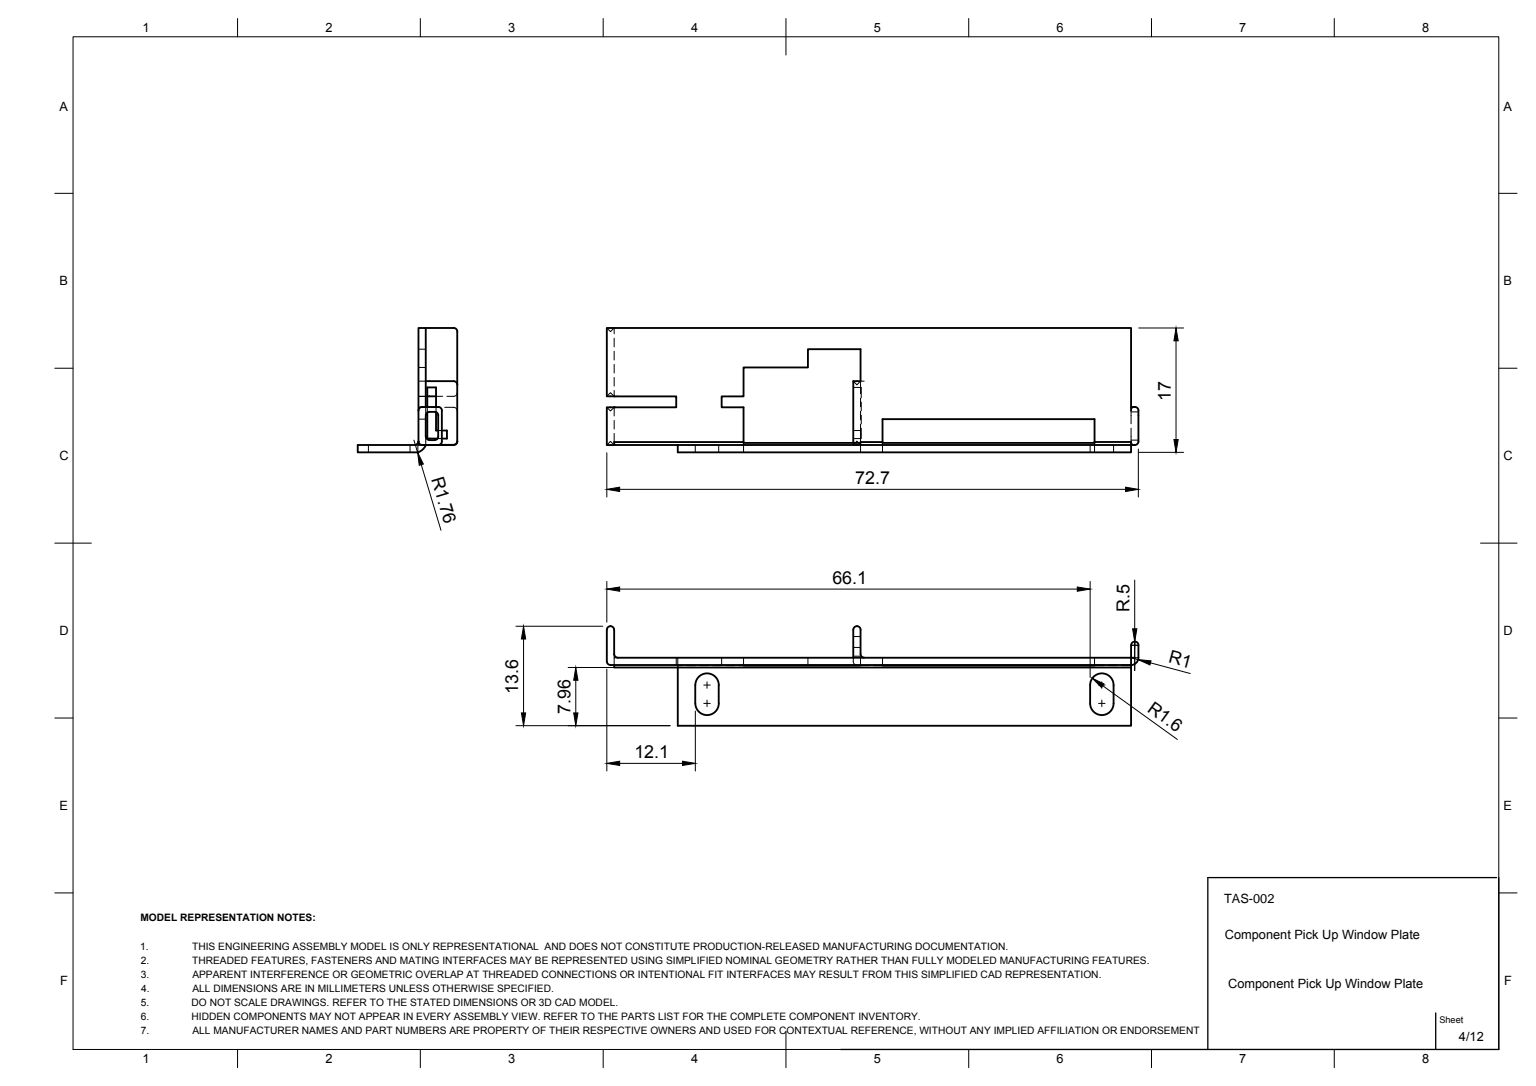
ISO-10303-21;
HEADER;
/* Generated by software containing ST-Developer
 * from STEP Tools, Inc. (www.steptools.com) 
 */

FILE_DESCRIPTION(
/* description */ ('STEP AP214'),
/* implementation_level */ '2;1');

FILE_NAME(
/* name */ 'Component Pick Up Window Plate.step',
/* time_stamp */ '2026-11-04T19:38:14-08:00',
/* author */ (''),
/* organization */ (''),
/* preprocessor_version */ 'ST-DEVELOPER v20.2',
/* originating_system */ 'Autodesk Translation Framework v15.17.0.0',
/* authorisation */ '');

FILE_SCHEMA (('AUTOMOTIVE_DESIGN { 1 0 10303 214 3 1 1 }'));
ENDSEC;

DATA;
#10=MECHANICAL_DESIGN_GEOMETRIC_PRESENTATION_REPRESENTATION('',(#471),#36668);
#385=SPHERICAL_SURFACE('',#18134,0.5);
#386=SPHERICAL_SURFACE('',#18138,0.5);
#407=(
BOUNDED_SURFACE()
B_SPLINE_SURFACE(2,2,((#25054,#25055,#25056),(#25057,#25058,#25059),(#25060,
#25061,#25062)),.UNSPECIFIED.,.F.,.F.,.F.)
B_SPLINE_SURFACE_WITH_KNOTS((3,3),(3,3),(-1.57079632679491,1.51262184115385E-31),
(-3.14159265358979,-1.57079632679489),.UNSPECIFIED.)
GEOMETRIC_REPRESENTATION_ITEM()
RATIONAL_B_SPLINE_SURFACE(((1.,0.707106781186547,1.),(0.707106781186636,
0.500000000000062,0.707106781186636),(1.,0.707106781186547,1.)))
REPRESENTATION_ITEM('')
SURFACE()
);
#408=(
BOUNDED_SURFACE()
B_SPLINE_SURFACE(2,2,((#25105,#25106,#25107),(#25108,#25109,#25110),(#25111,
#25112,#25113)),.UNSPECIFIED.,.F.,.F.,.F.)
B_SPLINE_SURFACE_WITH_KNOTS((3,3),(3,3),(-1.5707963267949,4.00000000000002E-15),
(-1.5707963267949,8.88178419700128E-15),.UNSPECIFIED.)
GEOMETRIC_REPRESENTATION_ITEM()
RATIONAL_B_SPLINE_SURFACE(((1.,0.707106781186544,1.),(0.707106781186621,
0.50000000000005,0.707106781186621),(1.,0.707106781186544,1.)))
REPRESENTATION_ITEM('')
SURFACE()
);
#417=ELLIPSE('',#18107,0.707106781183618,0.499999999997816);
#418=ELLIPSE('',#18108,0.70710678118541,0.499999999999275);
#419=ELLIPSE('',#18109,0.707106781187129,0.500000000000412);
#420=ELLIPSE('',#18110,0.707106781186662,0.500000000000074);
#421=ELLIPSE('',#18114,0.707106781185328,0.499999999999127);
#422=ELLIPSE('',#18115,0.707106781186805,0.500000000000239);
#423=ELLIPSE('',#18116,0.707106781186168,0.499999999999746);
#424=ELLIPSE('',#18117,0.707106781186428,0.499999999999895);
#425=ELLIPSE('',#18121,0.707106781186371,0.500000000000029);
#426=ELLIPSE('',#18122,0.707106781185591,0.499999999999375);
#427=ELLIPSE('',#18123,0.707106781187582,0.500000000000786);
#428=ELLIPSE('',#18124,0.707106781187168,0.500000000000398);
#451=SHAPE_REPRESENTATION_RELATIONSHIP('SRR','None',#36707,#461);
#461=ADVANCED_BREP_SHAPE_REPRESENTATION('',(#481),#36659);
#471=STYLED_ITEM('',(#36766),#481);
#481=MANIFOLD_SOLID_BREP('Body1',#17794);
#515=CYLINDRICAL_SURFACE('',#18106,0.5);
#516=CYLINDRICAL_SURFACE('',#18111,0.5);
#517=CYLINDRICAL_SURFACE('',#18112,0.5);
#518=CYLINDRICAL_SURFACE('',#18113,0.5);
#519=CYLINDRICAL_SURFACE('',#18118,0.5);
#520=CYLINDRICAL_SURFACE('',#18119,0.5);
#521=CYLINDRICAL_SURFACE('',#18120,0.5);
#522=CYLINDRICAL_SURFACE('',#18125,0.5);
#523=CYLINDRICAL_SURFACE('',#18126,0.5);
#524=CYLINDRICAL_SURFACE('',#18131,0.5);
#525=CYLINDRICAL_SURFACE('',#18136,0.5);
#526=CYLINDRICAL_SURFACE('',#18140,0.5);
#527=CYLINDRICAL_SURFACE('',#18147,0.5);
#528=CYLINDRICAL_SURFACE('',#18157,0.5);
#529=CYLINDRICAL_SURFACE('',#18160,0.5);
#530=CYLINDRICAL_SURFACE('',#18167,0.5);
#531=CYLINDRICAL_SURFACE('',#18170,0.5);
#532=CYLINDRICAL_SURFACE('',#18173,0.5);
#533=CYLINDRICAL_SURFACE('',#18176,0.5);
#534=CYLINDRICAL_SURFACE('',#18197,0.5);
#535=CYLINDRICAL_SURFACE('',#18200,0.5);
#536=CYLINDRICAL_SURFACE('',#18203,0.5);
#537=CYLINDRICAL_SURFACE('',#18206,0.5);
#538=CYLINDRICAL_SURFACE('',#18209,1.);
#539=CYLINDRICAL_SURFACE('',#18231,1.6);
#540=CYLINDRICAL_SURFACE('',#18235,1.6);
#541=CYLINDRICAL_SURFACE('',#18239,1.6);
#542=CYLINDRICAL_SURFACE('',#18243,1.6);
#543=CYLINDRICAL_SURFACE('',#18253,2.15235845279182);
#544=CYLINDRICAL_SURFACE('',#18258,1.76114216495771);
#545=CYLINDRICAL_SURFACE('',#18261,1.76114216495771);
#546=CYLINDRICAL_SURFACE('',#18262,1.76114216495771);
#880=FACE_BOUND('',#2725,.T.);
#881=FACE_BOUND('',#2780,.T.);
#882=FACE_BOUND('',#2781,.T.);
#883=FACE_BOUND('',#2788,.T.);
#884=FACE_BOUND('',#2789,.T.);
#1025=CIRCLE('',#18127,0.5);
#1026=CIRCLE('',#18128,1.);
#1027=CIRCLE('',#18129,0.5);
#1028=CIRCLE('',#18130,0.5);
#1029=CIRCLE('',#18132,0.5);
#1030=CIRCLE('',#18133,0.5);
#1031=CIRCLE('',#18135,0.5);
#1032=CIRCLE('',#18137,0.5);
#1033=CIRCLE('',#18139,0.5);
#1034=CIRCLE('',#18141,0.5);
#1035=CIRCLE('',#18142,0.5);
#1036=CIRCLE('',#18143,0.5);
#1037=CIRCLE('',#18144,0.5);
#1038=CIRCLE('',#18145,0.5);
#1039=CIRCLE('',#18146,1.);
#1040=CIRCLE('',#18148,0.5);
#1041=CIRCLE('',#18150,0.5);
#1042=CIRCLE('',#18155,0.5);
#1043=CIRCLE('',#18158,0.5);
#1044=CIRCLE('',#18159,0.5);
#1045=CIRCLE('',#18161,0.5);
#1046=CIRCLE('',#18162,0.5);
#1047=CIRCLE('',#18168,0.5);
#1048=CIRCLE('',#18169,0.5);
#1049=CIRCLE('',#18171,0.5);
#1050=CIRCLE('',#18172,0.5);
#1051=CIRCLE('',#18174,0.5);
#1052=CIRCLE('',#18175,0.5);
#1053=CIRCLE('',#18177,0.5);
#1054=CIRCLE('',#18178,0.5);
#1055=CIRCLE('',#18198,0.5);
#1056=CIRCLE('',#18199,0.5);
#1057=CIRCLE('',#18201,0.5);
#1058=CIRCLE('',#18202,0.5);
#1059=CIRCLE('',#18204,0.5);
#1060=CIRCLE('',#18205,0.5);
#1061=CIRCLE('',#18207,0.5);
#1062=CIRCLE('',#18208,0.5);
#1063=CIRCLE('',#18219,1.76114216495771);
#1064=CIRCLE('',#18220,2.15235845279182);
#1065=CIRCLE('',#18222,2.15235845279183);
#1066=CIRCLE('',#18223,1.76114216495771);
#1067=CIRCLE('',#18226,1.76114216495771);
#1068=CIRCLE('',#18227,2.15235845279182);
#1069=CIRCLE('',#18229,1.76114216495771);
#1070=CIRCLE('',#18230,2.15235845279182);
#1071=CIRCLE('',#18232,1.6);
#1072=CIRCLE('',#18233,1.6);
#1073=CIRCLE('',#18236,1.6);
#1074=CIRCLE('',#18237,1.6);
#1075=CIRCLE('',#18240,1.6);
#1076=CIRCLE('',#18241,1.6);
#1077=CIRCLE('',#18244,1.6);
#1078=CIRCLE('',#18245,1.6);
#1079=CIRCLE('',#18248,1.76114216495771);
#1080=CIRCLE('',#18251,2.15235845279182);
#1081=CIRCLE('',#18254,2.15235845279182);
#1082=CIRCLE('',#18263,1.76114216495771);
#1663=FACE_OUTER_BOUND('',#2698,.T.);
#1664=FACE_OUTER_BOUND('',#2699,.T.);
#1665=FACE_OUTER_BOUND('',#2700,.T.);
#1666=FACE_OUTER_BOUND('',#2701,.T.);
#1667=FACE_OUTER_BOUND('',#2702,.T.);
#1668=FACE_OUTER_BOUND('',#2703,.T.);
#1669=FACE_OUTER_BOUND('',#2704,.T.);
#1670=FACE_OUTER_BOUND('',#2705,.T.);
#1671=FACE_OUTER_BOUND('',#2706,.T.);
#1672=FACE_OUTER_BOUND('',#2707,.T.);
#1673=FACE_OUTER_BOUND('',#2708,.T.);
#1674=FACE_OUTER_BOUND('',#2709,.T.);
#1675=FACE_OUTER_BOUND('',#2710,.T.);
#1676=FACE_OUTER_BOUND('',#2711,.T.);
#1677=FACE_OUTER_BOUND('',#2712,.T.);
#1678=FACE_OUTER_BOUND('',#2713,.T.);
#1679=FACE_OUTER_BOUND('',#2714,.T.);
#1680=FACE_OUTER_BOUND('',#2715,.T.);
#1681=FACE_OUTER_BOUND('',#2716,.T.);
#1682=FACE_OUTER_BOUND('',#2717,.T.);
#1683=FACE_OUTER_BOUND('',#2718,.T.);
#1684=FACE_OUTER_BOUND('',#2719,.T.);
#1685=FACE_OUTER_BOUND('',#2720,.T.);
#1686=FACE_OUTER_BOUND('',#2721,.T.);
#1687=FACE_OUTER_BOUND('',#2722,.T.);
#1688=FACE_OUTER_BOUND('',#2723,.T.);
#1689=FACE_OUTER_BOUND('',#2724,.T.);
#1690=FACE_OUTER_BOUND('',#2726,.T.);
#1691=FACE_OUTER_BOUND('',#2727,.T.);
#1692=FACE_OUTER_BOUND('',#2728,.T.);
#1693=FACE_OUTER_BOUND('',#2729,.T.);
#1694=FACE_OUTER_BOUND('',#2730,.T.);
#1695=FACE_OUTER_BOUND('',#2731,.T.);
#1696=FACE_OUTER_BOUND('',#2732,.T.);
#1697=FACE_OUTER_BOUND('',#2733,.T.);
#1698=FACE_OUTER_BOUND('',#2734,.T.);
#1699=FACE_OUTER_BOUND('',#2735,.T.);
#1700=FACE_OUTER_BOUND('',#2736,.T.);
#1701=FACE_OUTER_BOUND('',#2737,.T.);
#1702=FACE_OUTER_BOUND('',#2738,.T.);
#1703=FACE_OUTER_BOUND('',#2739,.T.);
#1704=FACE_OUTER_BOUND('',#2740,.T.);
#1705=FACE_OUTER_BOUND('',#2741,.T.);
#1706=FACE_OUTER_BOUND('',#2742,.T.);
#1707=FACE_OUTER_BOUND('',#2743,.T.);
#1708=FACE_OUTER_BOUND('',#2744,.T.);
#1709=FACE_OUTER_BOUND('',#2745,.T.);
#1710=FACE_OUTER_BOUND('',#2746,.T.);
#1711=FACE_OUTER_BOUND('',#2747,.T.);
#1712=FACE_OUTER_BOUND('',#2748,.T.);
#1713=FACE_OUTER_BOUND('',#2749,.T.);
#1714=FACE_OUTER_BOUND('',#2750,.T.);
#1715=FACE_OUTER_BOUND('',#2751,.T.);
#1716=FACE_OUTER_BOUND('',#2752,.T.);
#1717=FACE_OUTER_BOUND('',#2753,.T.);
#1718=FACE_OUTER_BOUND('',#2754,.T.);
#1719=FACE_OUTER_BOUND('',#2755,.T.);
#1720=FACE_OUTER_BOUND('',#2756,.T.);
#1721=FACE_OUTER_BOUND('',#2757,.T.);
#1722=FACE_OUTER_BOUND('',#2758,.T.);
#1723=FACE_OUTER_BOUND('',#2759,.T.);
#1724=FACE_OUTER_BOUND('',#2760,.T.);
#1725=FACE_OUTER_BOUND('',#2761,.T.);
#1726=FACE_OUTER_BOUND('',#2762,.T.);
#1727=FACE_OUTER_BOUND('',#2763,.T.);
#1728=FACE_OUTER_BOUND('',#2764,.T.);
#1729=FACE_OUTER_BOUND('',#2765,.T.);
#1730=FACE_OUTER_BOUND('',#2766,.T.);
#1731=FACE_OUTER_BOUND('',#2767,.T.);
#1732=FACE_OUTER_BOUND('',#2768,.T.);
#1733=FACE_OUTER_BOUND('',#2769,.T.);
#1734=FACE_OUTER_BOUND('',#2770,.T.);
#1735=FACE_OUTER_BOUND('',#2771,.T.);
#1736=FACE_OUTER_BOUND('',#2772,.T.);
#1737=FACE_OUTER_BOUND('',#2773,.T.);
#1738=FACE_OUTER_BOUND('',#2774,.T.);
#1739=FACE_OUTER_BOUND('',#2775,.T.);
#1740=FACE_OUTER_BOUND('',#2776,.T.);
#1741=FACE_OUTER_BOUND('',#2777,.T.);
#1742=FACE_OUTER_BOUND('',#2778,.T.);
#1743=FACE_OUTER_BOUND('',#2779,.T.);
#1744=FACE_OUTER_BOUND('',#2782,.T.);
#1745=FACE_OUTER_BOUND('',#2783,.T.);
#1746=FACE_OUTER_BOUND('',#2784,.T.);
#1747=FACE_OUTER_BOUND('',#2785,.T.);
#1748=FACE_OUTER_BOUND('',#2786,.T.);
#1749=FACE_OUTER_BOUND('',#2787,.T.);
#1750=FACE_OUTER_BOUND('',#2790,.T.);
#1751=FACE_OUTER_BOUND('',#2791,.T.);
#1752=FACE_OUTER_BOUND('',#2792,.T.);
#1753=FACE_OUTER_BOUND('',#2793,.T.);
#1754=FACE_OUTER_BOUND('',#2794,.T.);
#1755=FACE_OUTER_BOUND('',#2795,.T.);
#1756=FACE_OUTER_BOUND('',#2796,.T.);
#1757=FACE_OUTER_BOUND('',#2797,.T.);
#1758=FACE_OUTER_BOUND('',#2798,.T.);
#2698=EDGE_LOOP('',(#12018,#12019,#12020,#12021,#12022,#12023));
#2699=EDGE_LOOP('',(#12024,#12025,#12026));
#2700=EDGE_LOOP('',(#12027,#12028,#12029));
#2701=EDGE_LOOP('',(#12030,#12031,#12032,#12033,#12034,#12035));
#2702=EDGE_LOOP('',(#12036,#12037,#12038));
#2703=EDGE_LOOP('',(#12039,#12040,#12041));
#2704=EDGE_LOOP('',(#12042,#12043,#12044,#12045,#12046,#12047));
#2705=EDGE_LOOP('',(#12048,#12049,#12050));
#2706=EDGE_LOOP('',(#12051,#12052,#12053));
#2707=EDGE_LOOP('',(#12054,#12055,#12056,#12057));
#2708=EDGE_LOOP('',(#12058,#12059,#12060,#12061,#12062));
#2709=EDGE_LOOP('',(#12063,#12064));
#2710=EDGE_LOOP('',(#12065,#12066,#12067,#12068,#12069,#12070,#12071,#12072));
#2711=EDGE_LOOP('',(#12073,#12074));
#2712=EDGE_LOOP('',(#12075,#12076,#12077,#12078,#12079));
#2713=EDGE_LOOP('',(#12080,#12081,#12082,#12083,#12084));
#2714=EDGE_LOOP('',(#12085,#12086,#12087,#12088));
#2715=EDGE_LOOP('',(#12089,#12090,#12091,#12092,#12093));
#2716=EDGE_LOOP('',(#12094,#12095,#12096,#12097));
#2717=EDGE_LOOP('',(#12098,#12099,#12100,#12101));
#2718=EDGE_LOOP('',(#12102,#12103,#12104,#12105));
#2719=EDGE_LOOP('',(#12106,#12107,#12108,#12109,#12110));
#2720=EDGE_LOOP('',(#12111,#12112,#12113,#12114));
#2721=EDGE_LOOP('',(#12115,#12116,#12117,#12118));
#2722=EDGE_LOOP('',(#12119,#12120,#12121,#12122,#12123,#12124,#12125,#12126));
#2723=EDGE_LOOP('',(#12127,#12128,#12129,#12130,#12131,#12132,#12133,#12134));
#2724=EDGE_LOOP('',(#12135,#12136,#12137,#12138));
#2725=EDGE_LOOP('',(#12139,#12140,#12141,#12142,#12143,#12144));
#2726=EDGE_LOOP('',(#12145,#12146,#12147,#12148,#12149,#12150,#12151,#12152));
#2727=EDGE_LOOP('',(#12153,#12154,#12155,#12156,#12157,#12158,#12159,#12160,
#12161,#12162));
#2728=EDGE_LOOP('',(#12163,#12164,#12165,#12166));
#2729=EDGE_LOOP('',(#12167,#12168,#12169,#12170));
#2730=EDGE_LOOP('',(#12171,#12172,#12173,#12174));
#2731=EDGE_LOOP('',(#12175,#12176,#12177,#12178));
#2732=EDGE_LOOP('',(#12179,#12180,#12181,#12182));
#2733=EDGE_LOOP('',(#12183,#12184,#12185,#12186));
#2734=EDGE_LOOP('',(#12187,#12188,#12189,#12190));
#2735=EDGE_LOOP('',(#12191,#12192,#12193,#12194));
#2736=EDGE_LOOP('',(#12195,#12196,#12197,#12198));
#2737=EDGE_LOOP('',(#12199,#12200,#12201,#12202));
#2738=EDGE_LOOP('',(#12203,#12204,#12205,#12206));
#2739=EDGE_LOOP('',(#12207,#12208,#12209,#12210));
#2740=EDGE_LOOP('',(#12211,#12212,#12213,#12214));
#2741=EDGE_LOOP('',(#12215,#12216,#12217,#12218,#12219));
#2742=EDGE_LOOP('',(#12220,#12221,#12222,#12223));
#2743=EDGE_LOOP('',(#12224,#12225,#12226,#12227));
#2744=EDGE_LOOP('',(#12228,#12229,#12230,#12231));
#2745=EDGE_LOOP('',(#12232,#12233,#12234,#12235,#12236,#12237,#12238,#12239));
#2746=EDGE_LOOP('',(#12240,#12241,#12242,#12243,#12244));
#2747=EDGE_LOOP('',(#12245,#12246,#12247,#12248));
#2748=EDGE_LOOP('',(#12249,#12250,#12251,#12252,#12253));
#2749=EDGE_LOOP('',(#12254,#12255,#12256,#12257,#12258,#12259,#12260,#12261));
#2750=EDGE_LOOP('',(#12262,#12263,#12264,#12265));
#2751=EDGE_LOOP('',(#12266,#12267,#12268,#12269));
#2752=EDGE_LOOP('',(#12270,#12271,#12272,#12273));
#2753=EDGE_LOOP('',(#12274,#12275,#12276,#12277));
#2754=EDGE_LOOP('',(#12278,#12279,#12280,#12281,#12282,#12283));
#2755=EDGE_LOOP('',(#12284,#12285,#12286,#12287));
#2756=EDGE_LOOP('',(#12288,#12289,#12290,#12291));
#2757=EDGE_LOOP('',(#12292,#12293,#12294,#12295));
#2758=EDGE_LOOP('',(#12296,#12297,#12298,#12299,#12300,#12301));
#2759=EDGE_LOOP('',(#12302,#12303,#12304,#12305,#12306,#12307));
#2760=EDGE_LOOP('',(#12308,#12309,#12310));
#2761=EDGE_LOOP('',(#12311,#12312,#12313));
#2762=EDGE_LOOP('',(#12314,#12315,#12316,#12317));
#2763=EDGE_LOOP('',(#12318,#12319,#12320,#12321,#12322,#12323));
#2764=EDGE_LOOP('',(#12324,#12325,#12326,#12327,#12328,#12329,#12330));
#2765=EDGE_LOOP('',(#12331,#12332,#12333,#12334));
#2766=EDGE_LOOP('',(#12335,#12336,#12337,#12338,#12339,#12340));
#2767=EDGE_LOOP('',(#12341,#12342,#12343,#12344,#12345,#12346));
#2768=EDGE_LOOP('',(#12347,#12348,#12349,#12350));
#2769=EDGE_LOOP('',(#12351,#12352,#12353,#12354));
#2770=EDGE_LOOP('',(#12355,#12356,#12357,#12358));
#2771=EDGE_LOOP('',(#12359,#12360,#12361,#12362));
#2772=EDGE_LOOP('',(#12363,#12364,#12365,#12366));
#2773=EDGE_LOOP('',(#12367,#12368,#12369,#12370));
#2774=EDGE_LOOP('',(#12371,#12372,#12373,#12374));
#2775=EDGE_LOOP('',(#12375,#12376,#12377,#12378));
#2776=EDGE_LOOP('',(#12379,#12380,#12381,#12382,#12383));
#2777=EDGE_LOOP('',(#12384,#12385,#12386,#12387,#12388,#12389));
#2778=EDGE_LOOP('',(#12390,#12391,#12392));
#2779=EDGE_LOOP('',(#12393,#12394,#12395,#12396));
#2780=EDGE_LOOP('',(#12397,#12398,#12399,#12400));
#2781=EDGE_LOOP('',(#12401,#12402,#12403,#12404));
#2782=EDGE_LOOP('',(#12405,#12406,#12407,#12408,#12409,#12410,#12411,#12412,
#12413,#12414,#12415,#12416,#12417));
#2783=EDGE_LOOP('',(#12418,#12419,#12420,#12421,#12422,#12423,#12424,#12425,
#12426,#12427,#12428,#12429,#12430,#12431,#12432,#12433,#12434,#12435,#12436,
#12437,#12438,#12439,#12440,#12441,#12442,#12443,#12444,#12445,#12446,#12447,
#12448,#12449,#12450,#12451));
#2784=EDGE_LOOP('',(#12452,#12453,#12454,#12455,#12456,#12457,#12458,#12459));
#2785=EDGE_LOOP('',(#12460,#12461,#12462,#12463,#12464,#12465,#12466,#12467,
#12468,#12469,#12470,#12471,#12472,#12473,#12474,#12475,#12476,#12477,#12478,
#12479,#12480,#12481,#12482,#12483,#12484,#12485,#12486,#12487,#12488,#12489,
#12490,#12491,#12492,#12493,#12494,#12495,#12496,#12497));
#2786=EDGE_LOOP('',(#12498,#12499,#12500,#12501));
#2787=EDGE_LOOP('',(#12502,#12503,#12504,#12505,#12506,#12507,#12508,#12509));
#2788=EDGE_LOOP('',(#12510,#12511,#12512,#12513));
#2789=EDGE_LOOP('',(#12514,#12515,#12516,#12517));
#2790=EDGE_LOOP('',(#12518,#12519,#12520,#12521));
#2791=EDGE_LOOP('',(#12522,#12523,#12524,#12525));
#2792=EDGE_LOOP('',(#12526,#12527,#12528,#12529));
#2793=EDGE_LOOP('',(#12530,#12531,#12532,#12533,#12534,#12535,#12536));
#2794=EDGE_LOOP('',(#12537,#12538,#12539,#12540,#12541));
#2795=EDGE_LOOP('',(#12542,#12543,#12544,#12545));
#2796=EDGE_LOOP('',(#12546,#12547,#12548,#12549));
#2797=EDGE_LOOP('',(#12550,#12551,#12552,#12553,#12554,#12555));
#2798=EDGE_LOOP('',(#12556,#12557,#12558,#12559,#12560,#12561));
#3936=LINE('',#25010,#5646);
#3937=LINE('',#25015,#5647);
#3938=LINE('',#25017,#5648);
#3939=LINE('',#25019,#5649);
#3940=LINE('',#25027,#5650);
#3941=LINE('',#25032,#5651);
#3942=LINE('',#25034,#5652);
#3943=LINE('',#25036,#5653);
#3944=LINE('',#25044,#5654);
#3945=LINE('',#25049,#5655);
#3946=LINE('',#25051,#5656);
#3947=LINE('',#25053,#5657);
#3948=LINE('',#25076,#5658);
#3949=LINE('',#25078,#5659);
#3950=LINE('',#25086,#5660);
#3951=LINE('',#25088,#5661);
#3952=LINE('',#25089,#5662);
#3953=LINE('',#25091,#5663);
#3954=LINE('',#25093,#5664);
#3955=LINE('',#25094,#5665);
#3956=LINE('',#25103,#5666);
#3957=LINE('',#25104,#5667);
#3958=LINE('',#25123,#5668);
#3959=LINE('',#25125,#5669);
#3960=LINE('',#25130,#5670);
#3961=LINE('',#25134,#5671);
#3962=LINE('',#25136,#5672);
#3963=LINE('',#25137,#5673);
#3964=LINE('',#25140,#5674);
#3965=LINE('',#25142,#5675);
#3966=LINE('',#25143,#5676);
#3967=LINE('',#25146,#5677);
#3968=LINE('',#25148,#5678);
#3969=LINE('',#25149,#5679);
#3970=LINE('',#25152,#5680);
#3971=LINE('',#25154,#5681);
#3972=LINE('',#25155,#5682);
#3973=LINE('',#25158,#5683);
#3974=LINE('',#25160,#5684);
#3975=LINE('',#25162,#5685);
#3976=LINE('',#25165,#5686);
#3977=LINE('',#25166,#5687);
#3978=LINE('',#25172,#5688);
#3979=LINE('',#25175,#5689);
#3980=LINE('',#25178,#5690);
#3981=LINE('',#25180,#5691);
#3982=LINE('',#25184,#5692);
#3983=LINE('',#25187,#5693);
#3984=LINE('',#25188,#5694);
#3985=LINE('',#25190,#5695);
#3986=LINE('',#25192,#5696);
#3987=LINE('',#25193,#5697);
#3988=LINE('',#25195,#5698);
#3989=LINE('',#25197,#5699);
#3990=LINE('',#25199,#5700);
#3991=LINE('',#25201,#5701);
#3992=LINE('',#25202,#5702);
#3993=LINE('',#25209,#5703);
#3994=LINE('',#25212,#5704);
#3995=LINE('',#25218,#5705);
#3996=LINE('',#25221,#5706);
#3997=LINE('',#25227,#5707);
#3998=LINE('',#25230,#5708);
#3999=LINE('',#25236,#5709);
#4000=LINE('',#25239,#5710);
#4001=LINE('',#25243,#5711);
#4002=LINE('',#25245,#5712);
#4003=LINE('',#25247,#5713);
#4004=LINE('',#25248,#5714);
#4005=LINE('',#25251,#5715);
#4006=LINE('',#25253,#5716);
#4007=LINE('',#25254,#5717);
#4008=LINE('',#25257,#5718);
#4009=LINE('',#25259,#5719);
#4010=LINE('',#25260,#5720);
#4011=LINE('',#25263,#5721);
#4012=LINE('',#25265,#5722);
#4013=LINE('',#25266,#5723);
#4014=LINE('',#25269,#5724);
#4015=LINE('',#25271,#5725);
#4016=LINE('',#25272,#5726);
#4017=LINE('',#25275,#5727);
#4018=LINE('',#25277,#5728);
#4019=LINE('',#25278,#5729);
#4020=LINE('',#25281,#5730);
#4021=LINE('',#25283,#5731);
#4022=LINE('',#25284,#5732);
#4023=LINE('',#25288,#5733);
#4024=LINE('',#25290,#5734);
#4025=LINE('',#25292,#5735);
#4026=LINE('',#25293,#5736);
#4027=LINE('',#25297,#5737);
#4028=LINE('',#25299,#5738);
#4029=LINE('',#25301,#5739);
#4030=LINE('',#25302,#5740);
#4031=LINE('',#25305,#5741);
#4032=LINE('',#25306,#5742);
#4033=LINE('',#25307,#5743);
#4034=LINE('',#25310,#5744);
#4035=LINE('',#25312,#5745);
#4036=LINE('',#25313,#5746);
#4037=LINE('',#25315,#5747);
#4038=LINE('',#25316,#5748);
#4039=LINE('',#25318,#5749);
#4040=LINE('',#25319,#5750);
#4041=LINE('',#25322,#5751);
#4042=LINE('',#25324,#5752);
#4043=LINE('',#25325,#5753);
#4044=LINE('',#25328,#5754);
#4045=LINE('',#25329,#5755);
#4046=LINE('',#25330,#5756);
#4047=LINE('',#25332,#5757);
#4048=LINE('',#25335,#5758);
#4049=LINE('',#25336,#5759);
#4050=LINE('',#25338,#5760);
#4051=LINE('',#25340,#5761);
#4052=LINE('',#25341,#5762);
#4053=LINE('',#25347,#5763);
#4054=LINE('',#25350,#5764);
#4055=LINE('',#25356,#5765);
#4056=LINE('',#25359,#5766);
#4057=LINE('',#25364,#5767);
#4058=LINE('',#25366,#5768);
#4059=LINE('',#25370,#5769);
#4060=LINE('',#25373,#5770);
#4061=LINE('',#25375,#5771);
#4062=LINE('',#25376,#5772);
#4063=LINE('',#25377,#5773);
#4064=LINE('',#25378,#5774);
#4065=LINE('',#25380,#5775);
#4066=LINE('',#25381,#5776);
#4067=LINE('',#25384,#5777);
#4068=LINE('',#25385,#5778);
#4069=LINE('',#25387,#5779);
#4070=LINE('',#25391,#5780);
#4071=LINE('',#25392,#5781);
#4072=LINE('',#25395,#5782);
#4073=LINE('',#25396,#5783);
#4074=LINE('',#25400,#5784);
#4075=LINE('',#25402,#5785);
#4076=LINE('',#25404,#5786);
#4077=LINE('',#25405,#5787);
#4078=LINE('',#25409,#5788);
#4079=LINE('',#25411,#5789);
#4080=LINE('',#25415,#5790);
#4081=LINE('',#25417,#5791);
#4082=LINE('',#25422,#5792);
#4083=LINE('',#25424,#5793);
#4084=LINE('',#25426,#5794);
#4085=LINE('',#25427,#5795);
#4086=LINE('',#25431,#5796);
#4087=LINE('',#25433,#5797);
#4088=LINE('',#25437,#5798);
#4089=LINE('',#25439,#5799);
#4090=LINE('',#25445,#5800);
#4091=LINE('',#25449,#5801);
#4092=LINE('',#25454,#5802);
#4093=LINE('',#25455,#5803);
#4094=LINE('',#25456,#5804);
#4095=LINE('',#25460,#5805);
#4096=LINE('',#25464,#5806);
#4097=LINE('',#25465,#5807);
#4098=LINE('',#25469,#5808);
#4099=LINE('',#25473,#5809);
#4100=LINE('',#25478,#5810);
#4101=LINE('',#25479,#5811);
#4102=LINE('',#25480,#5812);
#4103=LINE('',#25484,#5813);
#4104=LINE('',#25488,#5814);
#4105=LINE('',#25489,#5815);
#4106=LINE('',#25495,#5816);
#4107=LINE('',#25497,#5817);
#4108=LINE('',#25499,#5818);
#4109=LINE('',#25500,#5819);
#4110=LINE('',#25502,#5820);
#4111=LINE('',#25504,#5821);
#4112=LINE('',#25505,#5822);
#4113=LINE('',#25508,#5823);
#4114=LINE('',#25512,#5824);
#4115=LINE('',#25514,#5825);
#4116=LINE('',#25515,#5826);
#4117=LINE('',#25517,#5827);
#4118=LINE('',#25518,#5828);
#4119=LINE('',#25522,#5829);
#4120=LINE('',#25523,#5830);
#4121=LINE('',#25524,#5831);
#4122=LINE('',#25525,#5832);
#4123=LINE('',#25528,#5833);
#4124=LINE('',#25529,#5834);
#4125=LINE('',#25531,#5835);
#4126=LINE('',#25532,#5836);
#4127=LINE('',#25533,#5837);
#4128=LINE('',#25534,#5838);
#4129=LINE('',#25535,#5839);
#4130=LINE('',#25536,#5840);
#4131=LINE('',#25537,#5841);
#4132=LINE('',#25539,#5842);
#4133=LINE('',#25541,#5843);
#4134=LINE('',#25543,#5844);
#4135=LINE('',#25545,#5845);
#4136=LINE('',#25546,#5846);
#4137=LINE('',#25548,#5847);
#5646=VECTOR('',#20176,1000.);
#5647=VECTOR('',#20181,1000.);
#5648=VECTOR('',#20184,1000.);
#5649=VECTOR('',#20187,1000.);
#5650=VECTOR('',#20194,1000.);
#5651=VECTOR('',#20199,1000.);
#5652=VECTOR('',#20202,1000.);
#5653=VECTOR('',#20205,1000.);
#5654=VECTOR('',#20212,1000.);
#5655=VECTOR('',#20217,1000.);
#5656=VECTOR('',#20220,1000.);
#5657=VECTOR('',#20223,1000.);
#5658=VECTOR('',#20236,1000.);
#5659=VECTOR('',#20239,1000.);
#5660=VECTOR('',#20248,1000.);
#5661=VECTOR('',#20249,1000.);
#5662=VECTOR('',#20250,1000.);
#5663=VECTOR('',#20251,1000.);
#5664=VECTOR('',#20252,1000.);
#5665=VECTOR('',#20253,1000.);
#5666=VECTOR('',#20264,1000.);
#5667=VECTOR('',#20265,1000.);
#5668=VECTOR('',#20276,1000.);
#5669=VECTOR('',#20277,1000.);
#5670=VECTOR('',#20282,1000.);
#5671=VECTOR('',#20285,1000.);
#5672=VECTOR('',#20286,1000.);
#5673=VECTOR('',#20287,1000.);
#5674=VECTOR('',#20290,1000.);
#5675=VECTOR('',#20291,1000.);
#5676=VECTOR('',#20292,1000.);
#5677=VECTOR('',#20295,1000.);
#5678=VECTOR('',#20296,1000.);
#5679=VECTOR('',#20297,1000.);
#5680=VECTOR('',#20300,1000.);
#5681=VECTOR('',#20301,1000.);
#5682=VECTOR('',#20302,1000.);
#5683=VECTOR('',#20305,1000.);
#5684=VECTOR('',#20306,1000.);
#5685=VECTOR('',#20307,1000.);
#5686=VECTOR('',#20312,1000.);
#5687=VECTOR('',#20313,1000.);
#5688=VECTOR('',#20318,1000.);
#5689=VECTOR('',#20321,1000.);
#5690=VECTOR('',#20324,1000.);
#5691=VECTOR('',#20325,1000.);
#5692=VECTOR('',#20328,1000.);
#5693=VECTOR('',#20333,1000.);
#5694=VECTOR('',#20334,1000.);
#5695=VECTOR('',#20335,1000.);
#5696=VECTOR('',#20336,1000.);
#5697=VECTOR('',#20337,1000.);
#5698=VECTOR('',#20340,1000.);
#5699=VECTOR('',#20343,1000.);
#5700=VECTOR('',#20344,1000.);
#5701=VECTOR('',#20345,1000.);
#5702=VECTOR('',#20346,1000.);
#5703=VECTOR('',#20353,1000.);
#5704=VECTOR('',#20356,1000.);
#5705=VECTOR('',#20361,1000.);
#5706=VECTOR('',#20364,1000.);
#5707=VECTOR('',#20369,1000.);
#5708=VECTOR('',#20372,1000.);
#5709=VECTOR('',#20377,1000.);
#5710=VECTOR('',#20380,1000.);
#5711=VECTOR('',#20383,1000.);
#5712=VECTOR('',#20384,1000.);
#5713=VECTOR('',#20385,1000.);
#5714=VECTOR('',#20386,1000.);
#5715=VECTOR('',#20389,1000.);
#5716=VECTOR('',#20390,1000.);
#5717=VECTOR('',#20391,1000.);
#5718=VECTOR('',#20394,1000.);
#5719=VECTOR('',#20395,1000.);
#5720=VECTOR('',#20396,1000.);
#5721=VECTOR('',#20399,1000.);
#5722=VECTOR('',#20400,1000.);
#5723=VECTOR('',#20401,1000.);
#5724=VECTOR('',#20404,1000.);
#5725=VECTOR('',#20405,1000.);
#5726=VECTOR('',#20406,1000.);
#5727=VECTOR('',#20409,1000.);
#5728=VECTOR('',#20410,1000.);
#5729=VECTOR('',#20411,1000.);
#5730=VECTOR('',#20414,1000.);
#5731=VECTOR('',#20415,1000.);
#5732=VECTOR('',#20416,1000.);
#5733=VECTOR('',#20419,1000.);
#5734=VECTOR('',#20420,1000.);
#5735=VECTOR('',#20421,1000.);
#5736=VECTOR('',#20422,1000.);
#5737=VECTOR('',#20425,1000.);
#5738=VECTOR('',#20426,1000.);
#5739=VECTOR('',#20427,1000.);
#5740=VECTOR('',#20428,1000.);
#5741=VECTOR('',#20431,1000.);
#5742=VECTOR('',#20432,1000.);
#5743=VECTOR('',#20433,1000.);
#5744=VECTOR('',#20436,1000.);
#5745=VECTOR('',#20437,1000.);
#5746=VECTOR('',#20438,1000.);
#5747=VECTOR('',#20441,1000.);
#5748=VECTOR('',#20442,1000.);
#5749=VECTOR('',#20445,1000.);
#5750=VECTOR('',#20446,1000.);
#5751=VECTOR('',#20449,1000.);
#5752=VECTOR('',#20450,1000.);
#5753=VECTOR('',#20451,1000.);
#5754=VECTOR('',#20454,1000.);
#5755=VECTOR('',#20455,1000.);
#5756=VECTOR('',#20456,1000.);
#5757=VECTOR('',#20459,1000.);
#5758=VECTOR('',#20462,1000.);
#5759=VECTOR('',#20463,1000.);
#5760=VECTOR('',#20466,1000.);
#5761=VECTOR('',#20467,1000.);
#5762=VECTOR('',#20468,1000.);
#5763=VECTOR('',#20473,1000.);
#5764=VECTOR('',#20476,1000.);
#5765=VECTOR('',#20481,1000.);
#5766=VECTOR('',#20484,1000.);
#5767=VECTOR('',#20489,1000.);
#5768=VECTOR('',#20492,1000.);
#5769=VECTOR('',#20497,1000.);
#5770=VECTOR('',#20500,1000.);
#5771=VECTOR('',#20503,1000.);
#5772=VECTOR('',#20504,1000.);
#5773=VECTOR('',#20505,1000.);
#5774=VECTOR('',#20506,1000.);
#5775=VECTOR('',#20509,1000.);
#5776=VECTOR('',#20510,1000.);
#5777=VECTOR('',#20515,1000.);
#5778=VECTOR('',#20516,1000.);
#5779=VECTOR('',#20519,1000.);
#5780=VECTOR('',#20524,1000.);
#5781=VECTOR('',#20525,1000.);
#5782=VECTOR('',#20528,1000.);
#5783=VECTOR('',#20529,1000.);
#5784=VECTOR('',#20532,1000.);
#5785=VECTOR('',#20533,1000.);
#5786=VECTOR('',#20534,1000.);
#5787=VECTOR('',#20535,1000.);
#5788=VECTOR('',#20540,1000.);
#5789=VECTOR('',#20541,1000.);
#5790=VECTOR('',#20548,1000.);
#5791=VECTOR('',#20549,1000.);
#5792=VECTOR('',#20554,1000.);
#5793=VECTOR('',#20555,1000.);
#5794=VECTOR('',#20556,1000.);
#5795=VECTOR('',#20557,1000.);
#5796=VECTOR('',#20562,1000.);
#5797=VECTOR('',#20563,1000.);
#5798=VECTOR('',#20568,1000.);
#5799=VECTOR('',#20569,1000.);
#5800=VECTOR('',#20576,1000.);
#5801=VECTOR('',#20579,1000.);
#5802=VECTOR('',#20584,1000.);
#5803=VECTOR('',#20585,1000.);
#5804=VECTOR('',#20586,1000.);
#5805=VECTOR('',#20589,1000.);
#5806=VECTOR('',#20596,1000.);
#5807=VECTOR('',#20597,1000.);
#5808=VECTOR('',#20600,1000.);
#5809=VECTOR('',#20603,1000.);
#5810=VECTOR('',#20608,1000.);
#5811=VECTOR('',#20609,1000.);
#5812=VECTOR('',#20610,1000.);
#5813=VECTOR('',#20613,1000.);
#5814=VECTOR('',#20620,1000.);
#5815=VECTOR('',#20621,1000.);
#5816=VECTOR('',#20626,1000.);
#5817=VECTOR('',#20627,1000.);
#5818=VECTOR('',#20628,1000.);
#5819=VECTOR('',#20629,1000.);
#5820=VECTOR('',#20632,1000.);
#5821=VECTOR('',#20633,1000.);
#5822=VECTOR('',#20634,1000.);
#5823=VECTOR('',#20637,1000.);
#5824=VECTOR('',#20642,1000.);
#5825=VECTOR('',#20643,1000.);
#5826=VECTOR('',#20644,1000.);
#5827=VECTOR('',#20647,1000.);
#5828=VECTOR('',#20648,1000.);
#5829=VECTOR('',#20653,1000.);
#5830=VECTOR('',#20654,1000.);
#5831=VECTOR('',#20655,1000.);
#5832=VECTOR('',#20656,1000.);
#5833=VECTOR('',#20659,1000.);
#5834=VECTOR('',#20660,1000.);
#5835=VECTOR('',#20663,1000.);
#5836=VECTOR('',#20664,1000.);
#5837=VECTOR('',#20665,1000.);
#5838=VECTOR('',#20666,1000.);
#5839=VECTOR('',#20667,1000.);
#5840=VECTOR('',#20668,1000.);
#5841=VECTOR('',#20669,1000.);
#5842=VECTOR('',#20672,1000.);
#5843=VECTOR('',#20675,1000.);
#5844=VECTOR('',#20676,1000.);
#5845=VECTOR('',#20677,1000.);
#5846=VECTOR('',#20678,1000.);
#5847=VECTOR('',#20681,1000.);
#7274=VERTEX_POINT('',#25004);
#7275=VERTEX_POINT('',#25005);
#7276=VERTEX_POINT('',#25007);
#7277=VERTEX_POINT('',#25009);
#7278=VERTEX_POINT('',#25011);
#7279=VERTEX_POINT('',#25013);
#7280=VERTEX_POINT('',#25021);
#7281=VERTEX_POINT('',#25022);
#7282=VERTEX_POINT('',#25024);
#7283=VERTEX_POINT('',#25026);
#7284=VERTEX_POINT('',#25028);
#7285=VERTEX_POINT('',#25030);
#7286=VERTEX_POINT('',#25038);
#7287=VERTEX_POINT('',#25039);
#7288=VERTEX_POINT('',#25041);
#7289=VERTEX_POINT('',#25043);
#7290=VERTEX_POINT('',#25045);
#7291=VERTEX_POINT('',#25047);
#7292=VERTEX_POINT('',#25063);
#7293=VERTEX_POINT('',#25064);
#7294=VERTEX_POINT('',#25066);
#7295=VERTEX_POINT('',#25068);
#7296=VERTEX_POINT('',#25072);
#7297=VERTEX_POINT('',#25073);
#7298=VERTEX_POINT('',#25075);
#7299=VERTEX_POINT('',#25082);
#7300=VERTEX_POINT('',#25083);
#7301=VERTEX_POINT('',#25085);
#7302=VERTEX_POINT('',#25087);
#7303=VERTEX_POINT('',#25090);
#7304=VERTEX_POINT('',#25092);
#7305=VERTEX_POINT('',#25098);
#7306=VERTEX_POINT('',#25099);
#7307=VERTEX_POINT('',#25101);
#7308=VERTEX_POINT('',#25114);
#7309=VERTEX_POINT('',#25115);
#7310=VERTEX_POINT('',#25117);
#7311=VERTEX_POINT('',#25122);
#7312=VERTEX_POINT('',#25124);
#7313=VERTEX_POINT('',#25128);
#7314=VERTEX_POINT('',#25129);
#7315=VERTEX_POINT('',#25131);
#7316=VERTEX_POINT('',#25133);
#7317=VERTEX_POINT('',#25135);
#7318=VERTEX_POINT('',#25139);
#7319=VERTEX_POINT('',#25141);
#7320=VERTEX_POINT('',#25145);
#7321=VERTEX_POINT('',#25147);
#7322=VERTEX_POINT('',#25151);
#7323=VERTEX_POINT('',#25153);
#7324=VERTEX_POINT('',#25157);
#7325=VERTEX_POINT('',#25159);
#7326=VERTEX_POINT('',#25161);
#7327=VERTEX_POINT('',#25168);
#7328=VERTEX_POINT('',#25169);
#7329=VERTEX_POINT('',#25171);
#7330=VERTEX_POINT('',#25173);
#7331=VERTEX_POINT('',#25177);
#7332=VERTEX_POINT('',#25179);
#7333=VERTEX_POINT('',#25181);
#7334=VERTEX_POINT('',#25183);
#7335=VERTEX_POINT('',#25189);
#7336=VERTEX_POINT('',#25191);
#7337=VERTEX_POINT('',#25198);
#7338=VERTEX_POINT('',#25200);
#7339=VERTEX_POINT('',#25205);
#7340=VERTEX_POINT('',#25206);
#7341=VERTEX_POINT('',#25208);
#7342=VERTEX_POINT('',#25210);
#7343=VERTEX_POINT('',#25214);
#7344=VERTEX_POINT('',#25215);
#7345=VERTEX_POINT('',#25217);
#7346=VERTEX_POINT('',#25219);
#7347=VERTEX_POINT('',#25223);
#7348=VERTEX_POINT('',#25224);
#7349=VERTEX_POINT('',#25226);
#7350=VERTEX_POINT('',#25228);
#7351=VERTEX_POINT('',#25232);
#7352=VERTEX_POINT('',#25233);
#7353=VERTEX_POINT('',#25235);
#7354=VERTEX_POINT('',#25237);
#7355=VERTEX_POINT('',#25241);
#7356=VERTEX_POINT('',#25242);
#7357=VERTEX_POINT('',#25244);
#7358=VERTEX_POINT('',#25246);
#7359=VERTEX_POINT('',#25250);
#7360=VERTEX_POINT('',#25252);
#7361=VERTEX_POINT('',#25256);
#7362=VERTEX_POINT('',#25258);
#7363=VERTEX_POINT('',#25262);
#7364=VERTEX_POINT('',#25264);
#7365=VERTEX_POINT('',#25268);
#7366=VERTEX_POINT('',#25270);
#7367=VERTEX_POINT('',#25274);
#7368=VERTEX_POINT('',#25276);
#7369=VERTEX_POINT('',#25280);
#7370=VERTEX_POINT('',#25282);
#7371=VERTEX_POINT('',#25286);
#7372=VERTEX_POINT('',#25287);
#7373=VERTEX_POINT('',#25289);
#7374=VERTEX_POINT('',#25291);
#7375=VERTEX_POINT('',#25295);
#7376=VERTEX_POINT('',#25296);
#7377=VERTEX_POINT('',#25298);
#7378=VERTEX_POINT('',#25300);
#7379=VERTEX_POINT('',#25304);
#7380=VERTEX_POINT('',#25309);
#7381=VERTEX_POINT('',#25311);
#7382=VERTEX_POINT('',#25321);
#7383=VERTEX_POINT('',#25323);
#7384=VERTEX_POINT('',#25327);
#7385=VERTEX_POINT('',#25334);
#7386=VERTEX_POINT('',#25339);
#7387=VERTEX_POINT('',#25343);
#7388=VERTEX_POINT('',#25344);
#7389=VERTEX_POINT('',#25346);
#7390=VERTEX_POINT('',#25348);
#7391=VERTEX_POINT('',#25352);
#7392=VERTEX_POINT('',#25353);
#7393=VERTEX_POINT('',#25355);
#7394=VERTEX_POINT('',#25357);
#7395=VERTEX_POINT('',#25361);
#7396=VERTEX_POINT('',#25363);
#7397=VERTEX_POINT('',#25368);
#7398=VERTEX_POINT('',#25371);
#7399=VERTEX_POINT('',#25390);
#7400=VERTEX_POINT('',#25394);
#7401=VERTEX_POINT('',#25398);
#7402=VERTEX_POINT('',#25399);
#7403=VERTEX_POINT('',#25401);
#7404=VERTEX_POINT('',#25403);
#7405=VERTEX_POINT('',#25407);
#7406=VERTEX_POINT('',#25410);
#7407=VERTEX_POINT('',#25416);
#7408=VERTEX_POINT('',#25420);
#7409=VERTEX_POINT('',#25421);
#7410=VERTEX_POINT('',#25423);
#7411=VERTEX_POINT('',#25425);
#7412=VERTEX_POINT('',#25429);
#7413=VERTEX_POINT('',#25432);
#7414=VERTEX_POINT('',#25436);
#7415=VERTEX_POINT('',#25438);
#7416=VERTEX_POINT('',#25443);
#7417=VERTEX_POINT('',#25444);
#7418=VERTEX_POINT('',#25446);
#7419=VERTEX_POINT('',#25448);
#7420=VERTEX_POINT('',#25452);
#7421=VERTEX_POINT('',#25453);
#7422=VERTEX_POINT('',#25458);
#7423=VERTEX_POINT('',#25459);
#7424=VERTEX_POINT('',#25467);
#7425=VERTEX_POINT('',#25468);
#7426=VERTEX_POINT('',#25470);
#7427=VERTEX_POINT('',#25472);
#7428=VERTEX_POINT('',#25476);
#7429=VERTEX_POINT('',#25477);
#7430=VERTEX_POINT('',#25482);
#7431=VERTEX_POINT('',#25483);
#7432=VERTEX_POINT('',#25491);
#7433=VERTEX_POINT('',#25492);
#7434=VERTEX_POINT('',#25494);
#7435=VERTEX_POINT('',#25496);
#7436=VERTEX_POINT('',#25498);
#7437=VERTEX_POINT('',#25503);
#7438=VERTEX_POINT('',#25507);
#7439=VERTEX_POINT('',#25511);
#7440=VERTEX_POINT('',#25513);
#7441=VERTEX_POINT('',#25521);
#7442=VERTEX_POINT('',#25527);
#7443=VERTEX_POINT('',#25542);
#7444=VERTEX_POINT('',#25544);
#9061=EDGE_CURVE('',#7274,#7275,#417,.T.);
#9062=EDGE_CURVE('',#7276,#7275,#418,.T.);
#9063=EDGE_CURVE('',#7277,#7276,#3936,.T.);
#9064=EDGE_CURVE('',#7278,#7277,#419,.T.);
#9065=EDGE_CURVE('',#7278,#7279,#420,.T.);
#9066=EDGE_CURVE('',#7274,#7279,#3937,.T.);
#9067=EDGE_CURVE('',#7279,#7277,#3938,.T.);
#9068=EDGE_CURVE('',#7276,#7274,#3939,.T.);
#9069=EDGE_CURVE('',#7280,#7281,#421,.T.);
#9070=EDGE_CURVE('',#7282,#7281,#422,.T.);
#9071=EDGE_CURVE('',#7283,#7282,#3940,.T.);
#9072=EDGE_CURVE('',#7284,#7283,#423,.T.);
#9073=EDGE_CURVE('',#7284,#7285,#424,.T.);
#9074=EDGE_CURVE('',#7280,#7285,#3941,.T.);
#9075=EDGE_CURVE('',#7285,#7283,#3942,.T.);
#9076=EDGE_CURVE('',#7282,#7280,#3943,.T.);
#9077=EDGE_CURVE('',#7286,#7287,#425,.T.);
#9078=EDGE_CURVE('',#7288,#7287,#426,.T.);
#9079=EDGE_CURVE('',#7289,#7288,#3944,.T.);
#9080=EDGE_CURVE('',#7290,#7289,#427,.T.);
#9081=EDGE_CURVE('',#7290,#7291,#428,.T.);
#9082=EDGE_CURVE('',#7286,#7291,#3945,.T.);
#9083=EDGE_CURVE('',#7291,#7289,#3946,.T.);
#9084=EDGE_CURVE('',#7288,#7286,#3947,.T.);
#9085=EDGE_CURVE('',#7292,#7293,#1025,.T.);
#9086=EDGE_CURVE('',#7294,#7292,#1026,.T.);
#9087=EDGE_CURVE('',#7294,#7295,#1027,.T.);
#9088=EDGE_CURVE('',#7293,#7295,#1028,.T.);
#9089=EDGE_CURVE('',#7296,#7297,#1029,.T.);
#9090=EDGE_CURVE('',#7298,#7297,#3948,.T.);
#9091=EDGE_CURVE('',#7295,#7298,#1030,.T.);
#9092=EDGE_CURVE('',#7296,#7294,#3949,.T.);
#9093=EDGE_CURVE('',#7296,#7297,#1031,.T.);
#9094=EDGE_CURVE('',#7299,#7300,#1032,.T.);
#9095=EDGE_CURVE('',#7301,#7300,#3950,.T.);
#9096=EDGE_CURVE('',#7301,#7302,#3951,.T.);
#9097=EDGE_CURVE('',#7297,#7302,#3952,.T.);
#9098=EDGE_CURVE('',#7303,#7296,#3953,.T.);
#9099=EDGE_CURVE('',#7304,#7303,#3954,.T.);
#9100=EDGE_CURVE('',#7299,#7304,#3955,.T.);
#9101=EDGE_CURVE('',#7299,#7300,#1033,.T.);
#9102=EDGE_CURVE('',#7305,#7306,#1034,.T.);
#9103=EDGE_CURVE('',#7307,#7306,#1035,.T.);
#9104=EDGE_CURVE('',#7300,#7307,#3956,.T.);
#9105=EDGE_CURVE('',#7305,#7299,#3957,.T.);
#9106=EDGE_CURVE('',#7308,#7309,#1036,.T.);
#9107=EDGE_CURVE('',#7310,#7309,#1037,.T.);
#9108=EDGE_CURVE('',#7306,#7310,#1038,.T.);
#9109=EDGE_CURVE('',#7308,#7305,#1039,.T.);
#9110=EDGE_CURVE('',#7309,#7311,#3958,.T.);
#9111=EDGE_CURVE('',#7312,#7308,#3959,.T.);
#9112=EDGE_CURVE('',#7311,#7312,#1040,.T.);
#9113=EDGE_CURVE('',#7313,#7314,#3960,.T.);
#9114=EDGE_CURVE('',#7315,#7314,#1041,.T.);
#9115=EDGE_CURVE('',#7315,#7316,#3961,.T.);
#9116=EDGE_CURVE('',#7316,#7317,#3962,.T.);
#9117=EDGE_CURVE('',#7313,#7317,#3963,.T.);
#9118=EDGE_CURVE('',#7318,#7313,#3964,.T.);
#9119=EDGE_CURVE('',#7317,#7319,#3965,.T.);
#9120=EDGE_CURVE('',#7318,#7319,#3966,.T.);
#9121=EDGE_CURVE('',#7320,#7318,#3967,.T.);
#9122=EDGE_CURVE('',#7319,#7321,#3968,.T.);
#9123=EDGE_CURVE('',#7320,#7321,#3969,.T.);
#9124=EDGE_CURVE('',#7322,#7320,#3970,.T.);
#9125=EDGE_CURVE('',#7321,#7323,#3971,.T.);
#9126=EDGE_CURVE('',#7322,#7323,#3972,.T.);
#9127=EDGE_CURVE('',#7324,#7322,#3973,.T.);
#9128=EDGE_CURVE('',#7323,#7325,#3974,.T.);
#9129=EDGE_CURVE('',#7326,#7325,#3975,.T.);
#9130=EDGE_CURVE('',#7324,#7326,#1042,.T.);
#9131=EDGE_CURVE('',#7325,#7316,#3976,.T.);
#9132=EDGE_CURVE('',#7326,#7315,#3977,.T.);
#9133=EDGE_CURVE('',#7327,#7328,#1043,.T.);
#9134=EDGE_CURVE('',#7329,#7327,#3978,.T.);
#9135=EDGE_CURVE('',#7330,#7329,#1044,.T.);
#9136=EDGE_CURVE('',#7328,#7330,#3979,.T.);
#9137=EDGE_CURVE('',#7324,#7331,#3980,.T.);
#9138=EDGE_CURVE('',#7332,#7314,#3981,.T.);
#9139=EDGE_CURVE('',#7333,#7332,#1045,.T.);
#9140=EDGE_CURVE('',#7334,#7333,#3982,.T.);
#9141=EDGE_CURVE('',#7331,#7334,#1046,.T.);
#9142=EDGE_CURVE('',#7279,#7332,#3983,.T.);
#9143=EDGE_CURVE('',#7277,#7327,#3984,.T.);
#9144=EDGE_CURVE('',#7335,#7328,#3985,.T.);
#9145=EDGE_CURVE('',#7336,#7335,#3986,.T.);
#9146=EDGE_CURVE('',#7333,#7336,#3987,.T.);
#9147=EDGE_CURVE('',#7276,#7329,#3988,.T.);
#9148=EDGE_CURVE('',#7274,#7331,#3989,.T.);
#9149=EDGE_CURVE('',#7337,#7334,#3990,.T.);
#9150=EDGE_CURVE('',#7338,#7337,#3991,.T.);
#9151=EDGE_CURVE('',#7330,#7338,#3992,.T.);
#9152=EDGE_CURVE('',#7339,#7340,#1047,.T.);
#9153=EDGE_CURVE('',#7341,#7339,#3993,.T.);
#9154=EDGE_CURVE('',#7342,#7341,#1048,.T.);
#9155=EDGE_CURVE('',#7340,#7342,#3994,.T.);
#9156=EDGE_CURVE('',#7343,#7344,#1049,.T.);
#9157=EDGE_CURVE('',#7345,#7343,#3995,.T.);
#9158=EDGE_CURVE('',#7346,#7345,#1050,.T.);
#9159=EDGE_CURVE('',#7344,#7346,#3996,.T.);
#9160=EDGE_CURVE('',#7347,#7348,#1051,.T.);
#9161=EDGE_CURVE('',#7349,#7347,#3997,.T.);
#9162=EDGE_CURVE('',#7350,#7349,#1052,.T.);
#9163=EDGE_CURVE('',#7348,#7350,#3998,.T.);
#9164=EDGE_CURVE('',#7351,#7352,#1053,.T.);
#9165=EDGE_CURVE('',#7353,#7351,#3999,.T.);
#9166=EDGE_CURVE('',#7354,#7353,#1054,.T.);
#9167=EDGE_CURVE('',#7352,#7354,#4000,.T.);
#9168=EDGE_CURVE('',#7355,#7356,#4001,.T.);
#9169=EDGE_CURVE('',#7356,#7357,#4002,.T.);
#9170=EDGE_CURVE('',#7357,#7358,#4003,.T.);
#9171=EDGE_CURVE('',#7355,#7358,#4004,.T.);
#9172=EDGE_CURVE('',#7359,#7355,#4005,.T.);
#9173=EDGE_CURVE('',#7358,#7360,#4006,.T.);
#9174=EDGE_CURVE('',#7359,#7360,#4007,.T.);
#9175=EDGE_CURVE('',#7361,#7359,#4008,.T.);
#9176=EDGE_CURVE('',#7360,#7362,#4009,.T.);
#9177=EDGE_CURVE('',#7361,#7362,#4010,.T.);
#9178=EDGE_CURVE('',#7363,#7361,#4011,.T.);
#9179=EDGE_CURVE('',#7362,#7364,#4012,.T.);
#9180=EDGE_CURVE('',#7363,#7364,#4013,.T.);
#9181=EDGE_CURVE('',#7365,#7363,#4014,.T.);
#9182=EDGE_CURVE('',#7364,#7366,#4015,.T.);
#9183=EDGE_CURVE('',#7365,#7366,#4016,.T.);
#9184=EDGE_CURVE('',#7367,#7365,#4017,.T.);
#9185=EDGE_CURVE('',#7366,#7368,#4018,.T.);
#9186=EDGE_CURVE('',#7367,#7368,#4019,.T.);
#9187=EDGE_CURVE('',#7369,#7367,#4020,.T.);
#9188=EDGE_CURVE('',#7368,#7370,#4021,.T.);
#9189=EDGE_CURVE('',#7369,#7370,#4022,.T.);
#9190=EDGE_CURVE('',#7371,#7372,#4023,.T.);
#9191=EDGE_CURVE('',#7372,#7373,#4024,.T.);
#9192=EDGE_CURVE('',#7373,#7374,#4025,.T.);
#9193=EDGE_CURVE('',#7371,#7374,#4026,.T.);
#9194=EDGE_CURVE('',#7375,#7376,#4027,.T.);
#9195=EDGE_CURVE('',#7376,#7377,#4028,.T.);
#9196=EDGE_CURVE('',#7377,#7378,#4029,.T.);
#9197=EDGE_CURVE('',#7375,#7378,#4030,.T.);
#9198=EDGE_CURVE('',#7379,#7375,#4031,.T.);
#9199=EDGE_CURVE('',#7378,#7347,#4032,.T.);
#9200=EDGE_CURVE('',#7379,#7348,#4033,.T.);
#9201=EDGE_CURVE('',#7376,#7380,#4034,.T.);
#9202=EDGE_CURVE('',#7380,#7381,#4035,.T.);
#9203=EDGE_CURVE('',#7381,#7377,#4036,.T.);
#9204=EDGE_CURVE('',#7280,#7354,#4037,.T.);
#9205=EDGE_CURVE('',#7285,#7352,#4038,.T.);
#9206=EDGE_CURVE('',#7283,#7343,#4039,.T.);
#9207=EDGE_CURVE('',#7282,#7345,#4040,.T.);
#9208=EDGE_CURVE('',#7382,#7353,#4041,.T.);
#9209=EDGE_CURVE('',#7382,#7383,#4042,.T.);
#9210=EDGE_CURVE('',#7346,#7383,#4043,.T.);
#9211=EDGE_CURVE('',#7291,#7384,#4044,.T.);
#9212=EDGE_CURVE('',#7289,#7339,#4045,.T.);
#9213=EDGE_CURVE('',#7384,#7340,#4046,.T.);
#9214=EDGE_CURVE('',#7288,#7341,#4047,.T.);
#9215=EDGE_CURVE('',#7286,#7385,#4048,.T.);
#9216=EDGE_CURVE('',#7342,#7385,#4049,.T.);
#9217=EDGE_CURVE('',#7384,#7379,#4050,.T.);
#9218=EDGE_CURVE('',#7386,#7350,#4051,.T.);
#9219=EDGE_CURVE('',#7385,#7386,#4052,.T.);
#9220=EDGE_CURVE('',#7387,#7388,#1055,.T.);
#9221=EDGE_CURVE('',#7389,#7387,#4053,.T.);
#9222=EDGE_CURVE('',#7390,#7389,#1056,.T.);
#9223=EDGE_CURVE('',#7388,#7390,#4054,.T.);
#9224=EDGE_CURVE('',#7391,#7392,#1057,.T.);
#9225=EDGE_CURVE('',#7393,#7391,#4055,.T.);
#9226=EDGE_CURVE('',#7394,#7393,#1058,.T.);
#9227=EDGE_CURVE('',#7392,#7394,#4056,.T.);
#9228=EDGE_CURVE('',#7395,#7301,#1059,.T.);
#9229=EDGE_CURVE('',#7396,#7395,#4057,.T.);
#9230=EDGE_CURVE('',#7304,#7396,#1060,.T.);
#9231=EDGE_CURVE('',#7301,#7304,#4058,.T.);
#9232=EDGE_CURVE('',#7302,#7397,#1061,.T.);
#9233=EDGE_CURVE('',#7303,#7302,#4059,.T.);
#9234=EDGE_CURVE('',#7398,#7303,#1062,.T.);
#9235=EDGE_CURVE('',#7397,#7398,#4060,.T.);
#9236=EDGE_CURVE('',#7294,#7390,#4061,.T.);
#9237=EDGE_CURVE('',#7308,#7292,#4062,.T.);
#9238=EDGE_CURVE('',#7393,#7305,#4063,.T.);
#9239=EDGE_CURVE('',#7390,#7393,#4064,.T.);
#9240=EDGE_CURVE('',#7394,#7396,#4065,.T.);
#9241=EDGE_CURVE('',#7392,#7395,#4066,.T.);
#9242=EDGE_CURVE('',#7397,#7387,#4067,.T.);
#9243=EDGE_CURVE('',#7398,#7389,#4068,.T.);
#9244=EDGE_CURVE('',#7307,#7391,#4069,.T.);
#9245=EDGE_CURVE('',#7399,#7306,#4070,.T.);
#9246=EDGE_CURVE('',#7310,#7399,#4071,.T.);
#9247=EDGE_CURVE('',#7400,#7293,#4072,.T.);
#9248=EDGE_CURVE('',#7295,#7400,#4073,.T.);
#9249=EDGE_CURVE('',#7401,#7402,#4074,.T.);
#9250=EDGE_CURVE('',#7402,#7403,#4075,.T.);
#9251=EDGE_CURVE('',#7403,#7404,#4076,.T.);
#9252=EDGE_CURVE('',#7401,#7404,#4077,.T.);
#9253=EDGE_CURVE('',#7404,#7405,#1063,.T.);
#9254=EDGE_CURVE('',#7405,#7373,#4078,.T.);
#9255=EDGE_CURVE('',#7372,#7406,#4079,.T.);
#9256=EDGE_CURVE('',#7406,#7401,#1064,.T.);
#9257=EDGE_CURVE('',#7402,#7311,#1065,.T.);
#9258=EDGE_CURVE('',#7312,#7371,#4080,.T.);
#9259=EDGE_CURVE('',#7374,#7407,#4081,.T.);
#9260=EDGE_CURVE('',#7407,#7403,#1066,.T.);
#9261=EDGE_CURVE('',#7408,#7409,#4082,.T.);
#9262=EDGE_CURVE('',#7409,#7410,#4083,.T.);
#9263=EDGE_CURVE('',#7410,#7411,#4084,.T.);
#9264=EDGE_CURVE('',#7408,#7411,#4085,.T.);
#9265=EDGE_CURVE('',#7411,#7412,#1067,.T.);
#9266=EDGE_CURVE('',#7412,#7357,#4086,.T.);
#9267=EDGE_CURVE('',#7356,#7413,#4087,.T.);
#9268=EDGE_CURVE('',#7413,#7408,#1068,.T.);
#9269=EDGE_CURVE('',#7338,#7414,#4088,.T.);
#9270=EDGE_CURVE('',#7337,#7415,#4089,.T.);
#9271=EDGE_CURVE('',#7415,#7410,#1069,.T.);
#9272=EDGE_CURVE('',#7409,#7414,#1070,.T.);
#9273=EDGE_CURVE('',#7416,#7417,#4090,.T.);
#9274=EDGE_CURVE('',#7417,#7418,#1071,.T.);
#9275=EDGE_CURVE('',#7419,#7418,#4091,.T.);
#9276=EDGE_CURVE('',#7416,#7419,#1072,.T.);
#9277=EDGE_CURVE('',#7420,#7421,#4092,.T.);
#9278=EDGE_CURVE('',#7421,#7417,#4093,.T.);
#9279=EDGE_CURVE('',#7420,#7416,#4094,.T.);
#9280=EDGE_CURVE('',#7422,#7423,#4095,.T.);
#9281=EDGE_CURVE('',#7423,#7421,#1073,.T.);
#9282=EDGE_CURVE('',#7422,#7420,#1074,.T.);
#9283=EDGE_CURVE('',#7418,#7423,#4096,.T.);
#9284=EDGE_CURVE('',#7419,#7422,#4097,.T.);
#9285=EDGE_CURVE('',#7424,#7425,#4098,.T.);
#9286=EDGE_CURVE('',#7425,#7426,#1075,.T.);
#9287=EDGE_CURVE('',#7427,#7426,#4099,.T.);
#9288=EDGE_CURVE('',#7424,#7427,#1076,.T.);
#9289=EDGE_CURVE('',#7428,#7429,#4100,.T.);
#9290=EDGE_CURVE('',#7429,#7425,#4101,.T.);
#9291=EDGE_CURVE('',#7428,#7424,#4102,.T.);
#9292=EDGE_CURVE('',#7430,#7431,#4103,.T.);
#9293=EDGE_CURVE('',#7431,#7429,#1077,.T.);
#9294=EDGE_CURVE('',#7430,#7428,#1078,.T.);
#9295=EDGE_CURVE('',#7426,#7431,#4104,.T.);
#9296=EDGE_CURVE('',#7427,#7430,#4105,.T.);
#9297=EDGE_CURVE('',#7432,#7433,#1079,.T.);
#9298=EDGE_CURVE('',#7433,#7434,#4106,.T.);
#9299=EDGE_CURVE('',#7435,#7434,#4107,.T.);
#9300=EDGE_CURVE('',#7436,#7435,#4108,.T.);
#9301=EDGE_CURVE('',#7432,#7436,#4109,.T.);
#9302=EDGE_CURVE('',#7349,#7432,#4110,.T.);
#9303=EDGE_CURVE('',#7436,#7437,#4111,.T.);
#9304=EDGE_CURVE('',#7437,#7386,#4112,.T.);
#9305=EDGE_CURVE('',#7386,#7438,#4113,.T.);
#9306=EDGE_CURVE('',#7437,#7438,#1080,.T.);
#9307=EDGE_CURVE('',#7439,#7435,#4114,.T.);
#9308=EDGE_CURVE('',#7439,#7440,#4115,.T.);
#9309=EDGE_CURVE('',#7440,#7436,#4116,.T.);
#9310=EDGE_CURVE('',#7406,#7414,#4117,.T.);
#9311=EDGE_CURVE('',#7413,#7438,#4118,.T.);
#9312=EDGE_CURVE('',#7440,#7309,#1081,.T.);
#9313=EDGE_CURVE('',#7292,#7441,#4119,.T.);
#9314=EDGE_CURVE('',#7441,#7344,#4120,.T.);
#9315=EDGE_CURVE('',#7380,#7383,#4121,.T.);
#9316=EDGE_CURVE('',#7335,#7369,#4122,.T.);
#9317=EDGE_CURVE('',#7441,#7442,#4123,.T.);
#9318=EDGE_CURVE('',#7442,#7351,#4124,.T.);
#9319=EDGE_CURVE('',#7370,#7336,#4125,.T.);
#9320=EDGE_CURVE('',#7412,#7432,#4126,.T.);
#9321=EDGE_CURVE('',#7382,#7381,#4127,.T.);
#9322=EDGE_CURVE('',#7442,#7400,#4128,.T.);
#9323=EDGE_CURVE('',#7388,#7298,#4129,.T.);
#9324=EDGE_CURVE('',#7399,#7407,#4130,.T.);
#9325=EDGE_CURVE('',#7405,#7415,#4131,.T.);
#9326=EDGE_CURVE('',#7411,#7433,#4132,.T.);
#9327=EDGE_CURVE('',#7404,#7410,#4133,.T.);
#9328=EDGE_CURVE('',#7443,#7403,#4134,.T.);
#9329=EDGE_CURVE('',#7443,#7444,#4135,.T.);
#9330=EDGE_CURVE('',#7444,#7434,#4136,.T.);
#9331=EDGE_CURVE('',#7444,#7439,#4137,.T.);
#9332=EDGE_CURVE('',#7399,#7443,#1082,.T.);
#12018=ORIENTED_EDGE('',*,*,#9061,.T.);
#12019=ORIENTED_EDGE('',*,*,#9062,.F.);
#12020=ORIENTED_EDGE('',*,*,#9063,.F.);
#12021=ORIENTED_EDGE('',*,*,#9064,.F.);
#12022=ORIENTED_EDGE('',*,*,#9065,.T.);
#12023=ORIENTED_EDGE('',*,*,#9066,.F.);
#12024=ORIENTED_EDGE('',*,*,#9064,.T.);
#12025=ORIENTED_EDGE('',*,*,#9067,.F.);
#12026=ORIENTED_EDGE('',*,*,#9065,.F.);
#12027=ORIENTED_EDGE('',*,*,#9068,.F.);
#12028=ORIENTED_EDGE('',*,*,#9062,.T.);
#12029=ORIENTED_EDGE('',*,*,#9061,.F.);
#12030=ORIENTED_EDGE('',*,*,#9069,.T.);
#12031=ORIENTED_EDGE('',*,*,#9070,.F.);
#12032=ORIENTED_EDGE('',*,*,#9071,.F.);
#12033=ORIENTED_EDGE('',*,*,#9072,.F.);
#12034=ORIENTED_EDGE('',*,*,#9073,.T.);
#12035=ORIENTED_EDGE('',*,*,#9074,.F.);
#12036=ORIENTED_EDGE('',*,*,#9072,.T.);
#12037=ORIENTED_EDGE('',*,*,#9075,.F.);
#12038=ORIENTED_EDGE('',*,*,#9073,.F.);
#12039=ORIENTED_EDGE('',*,*,#9076,.F.);
#12040=ORIENTED_EDGE('',*,*,#9070,.T.);
#12041=ORIENTED_EDGE('',*,*,#9069,.F.);
#12042=ORIENTED_EDGE('',*,*,#9077,.T.);
#12043=ORIENTED_EDGE('',*,*,#9078,.F.);
#12044=ORIENTED_EDGE('',*,*,#9079,.F.);
#12045=ORIENTED_EDGE('',*,*,#9080,.F.);
#12046=ORIENTED_EDGE('',*,*,#9081,.T.);
#12047=ORIENTED_EDGE('',*,*,#9082,.F.);
#12048=ORIENTED_EDGE('',*,*,#9080,.T.);
#12049=ORIENTED_EDGE('',*,*,#9083,.F.);
#12050=ORIENTED_EDGE('',*,*,#9081,.F.);
#12051=ORIENTED_EDGE('',*,*,#9084,.F.);
#12052=ORIENTED_EDGE('',*,*,#9078,.T.);
#12053=ORIENTED_EDGE('',*,*,#9077,.F.);
#12054=ORIENTED_EDGE('',*,*,#9085,.F.);
#12055=ORIENTED_EDGE('',*,*,#9086,.F.);
#12056=ORIENTED_EDGE('',*,*,#9087,.T.);
#12057=ORIENTED_EDGE('',*,*,#9088,.F.);
#12058=ORIENTED_EDGE('',*,*,#9089,.T.);
#12059=ORIENTED_EDGE('',*,*,#9090,.F.);
#12060=ORIENTED_EDGE('',*,*,#9091,.F.);
#12061=ORIENTED_EDGE('',*,*,#9087,.F.);
#12062=ORIENTED_EDGE('',*,*,#9092,.F.);
#12063=ORIENTED_EDGE('',*,*,#9093,.T.);
#12064=ORIENTED_EDGE('',*,*,#9089,.F.);
#12065=ORIENTED_EDGE('',*,*,#9094,.T.);
#12066=ORIENTED_EDGE('',*,*,#9095,.F.);
#12067=ORIENTED_EDGE('',*,*,#9096,.T.);
#12068=ORIENTED_EDGE('',*,*,#9097,.F.);
#12069=ORIENTED_EDGE('',*,*,#9093,.F.);
#12070=ORIENTED_EDGE('',*,*,#9098,.F.);
#12071=ORIENTED_EDGE('',*,*,#9099,.F.);
#12072=ORIENTED_EDGE('',*,*,#9100,.F.);
#12073=ORIENTED_EDGE('',*,*,#9101,.T.);
#12074=ORIENTED_EDGE('',*,*,#9094,.F.);
#12075=ORIENTED_EDGE('',*,*,#9102,.T.);
#12076=ORIENTED_EDGE('',*,*,#9103,.F.);
#12077=ORIENTED_EDGE('',*,*,#9104,.F.);
#12078=ORIENTED_EDGE('',*,*,#9101,.F.);
#12079=ORIENTED_EDGE('',*,*,#9105,.F.);
#12080=ORIENTED_EDGE('',*,*,#9106,.T.);
#12081=ORIENTED_EDGE('',*,*,#9107,.F.);
#12082=ORIENTED_EDGE('',*,*,#9108,.F.);
#12083=ORIENTED_EDGE('',*,*,#9102,.F.);
#12084=ORIENTED_EDGE('',*,*,#9109,.F.);
#12085=ORIENTED_EDGE('',*,*,#9110,.F.);
#12086=ORIENTED_EDGE('',*,*,#9106,.F.);
#12087=ORIENTED_EDGE('',*,*,#9111,.F.);
#12088=ORIENTED_EDGE('',*,*,#9112,.F.);
#12089=ORIENTED_EDGE('',*,*,#9113,.T.);
#12090=ORIENTED_EDGE('',*,*,#9114,.F.);
#12091=ORIENTED_EDGE('',*,*,#9115,.T.);
#12092=ORIENTED_EDGE('',*,*,#9116,.T.);
#12093=ORIENTED_EDGE('',*,*,#9117,.F.);
#12094=ORIENTED_EDGE('',*,*,#9118,.T.);
#12095=ORIENTED_EDGE('',*,*,#9117,.T.);
#12096=ORIENTED_EDGE('',*,*,#9119,.T.);
#12097=ORIENTED_EDGE('',*,*,#9120,.F.);
#12098=ORIENTED_EDGE('',*,*,#9121,.T.);
#12099=ORIENTED_EDGE('',*,*,#9120,.T.);
#12100=ORIENTED_EDGE('',*,*,#9122,.T.);
#12101=ORIENTED_EDGE('',*,*,#9123,.F.);
#12102=ORIENTED_EDGE('',*,*,#9124,.T.);
#12103=ORIENTED_EDGE('',*,*,#9123,.T.);
#12104=ORIENTED_EDGE('',*,*,#9125,.T.);
#12105=ORIENTED_EDGE('',*,*,#9126,.F.);
#12106=ORIENTED_EDGE('',*,*,#9127,.T.);
#12107=ORIENTED_EDGE('',*,*,#9126,.T.);
#12108=ORIENTED_EDGE('',*,*,#9128,.T.);
#12109=ORIENTED_EDGE('',*,*,#9129,.F.);
#12110=ORIENTED_EDGE('',*,*,#9130,.F.);
#12111=ORIENTED_EDGE('',*,*,#9129,.T.);
#12112=ORIENTED_EDGE('',*,*,#9131,.T.);
#12113=ORIENTED_EDGE('',*,*,#9115,.F.);
#12114=ORIENTED_EDGE('',*,*,#9132,.F.);
#12115=ORIENTED_EDGE('',*,*,#9133,.F.);
#12116=ORIENTED_EDGE('',*,*,#9134,.F.);
#12117=ORIENTED_EDGE('',*,*,#9135,.F.);
#12118=ORIENTED_EDGE('',*,*,#9136,.F.);
#12119=ORIENTED_EDGE('',*,*,#9137,.F.);
#12120=ORIENTED_EDGE('',*,*,#9130,.T.);
#12121=ORIENTED_EDGE('',*,*,#9132,.T.);
#12122=ORIENTED_EDGE('',*,*,#9114,.T.);
#12123=ORIENTED_EDGE('',*,*,#9138,.F.);
#12124=ORIENTED_EDGE('',*,*,#9139,.F.);
#12125=ORIENTED_EDGE('',*,*,#9140,.F.);
#12126=ORIENTED_EDGE('',*,*,#9141,.F.);
#12127=ORIENTED_EDGE('',*,*,#9142,.F.);
#12128=ORIENTED_EDGE('',*,*,#9067,.T.);
#12129=ORIENTED_EDGE('',*,*,#9143,.T.);
#12130=ORIENTED_EDGE('',*,*,#9133,.T.);
#12131=ORIENTED_EDGE('',*,*,#9144,.F.);
#12132=ORIENTED_EDGE('',*,*,#9145,.F.);
#12133=ORIENTED_EDGE('',*,*,#9146,.F.);
#12134=ORIENTED_EDGE('',*,*,#9139,.T.);
#12135=ORIENTED_EDGE('',*,*,#9143,.F.);
#12136=ORIENTED_EDGE('',*,*,#9063,.T.);
#12137=ORIENTED_EDGE('',*,*,#9147,.T.);
#12138=ORIENTED_EDGE('',*,*,#9134,.T.);
#12139=ORIENTED_EDGE('',*,*,#9128,.F.);
#12140=ORIENTED_EDGE('',*,*,#9125,.F.);
#12141=ORIENTED_EDGE('',*,*,#9122,.F.);
#12142=ORIENTED_EDGE('',*,*,#9119,.F.);
#12143=ORIENTED_EDGE('',*,*,#9116,.F.);
#12144=ORIENTED_EDGE('',*,*,#9131,.F.);
#12145=ORIENTED_EDGE('',*,*,#9147,.F.);
#12146=ORIENTED_EDGE('',*,*,#9068,.T.);
#12147=ORIENTED_EDGE('',*,*,#9148,.T.);
#12148=ORIENTED_EDGE('',*,*,#9141,.T.);
#12149=ORIENTED_EDGE('',*,*,#9149,.F.);
#12150=ORIENTED_EDGE('',*,*,#9150,.F.);
#12151=ORIENTED_EDGE('',*,*,#9151,.F.);
#12152=ORIENTED_EDGE('',*,*,#9135,.T.);
#12153=ORIENTED_EDGE('',*,*,#9148,.F.);
#12154=ORIENTED_EDGE('',*,*,#9066,.T.);
#12155=ORIENTED_EDGE('',*,*,#9142,.T.);
#12156=ORIENTED_EDGE('',*,*,#9138,.T.);
#12157=ORIENTED_EDGE('',*,*,#9113,.F.);
#12158=ORIENTED_EDGE('',*,*,#9118,.F.);
#12159=ORIENTED_EDGE('',*,*,#9121,.F.);
#12160=ORIENTED_EDGE('',*,*,#9124,.F.);
#12161=ORIENTED_EDGE('',*,*,#9127,.F.);
#12162=ORIENTED_EDGE('',*,*,#9137,.T.);
#12163=ORIENTED_EDGE('',*,*,#9152,.F.);
#12164=ORIENTED_EDGE('',*,*,#9153,.F.);
#12165=ORIENTED_EDGE('',*,*,#9154,.F.);
#12166=ORIENTED_EDGE('',*,*,#9155,.F.);
#12167=ORIENTED_EDGE('',*,*,#9156,.F.);
#12168=ORIENTED_EDGE('',*,*,#9157,.F.);
#12169=ORIENTED_EDGE('',*,*,#9158,.F.);
#12170=ORIENTED_EDGE('',*,*,#9159,.F.);
#12171=ORIENTED_EDGE('',*,*,#9160,.F.);
#12172=ORIENTED_EDGE('',*,*,#9161,.F.);
#12173=ORIENTED_EDGE('',*,*,#9162,.F.);
#12174=ORIENTED_EDGE('',*,*,#9163,.F.);
#12175=ORIENTED_EDGE('',*,*,#9164,.F.);
#12176=ORIENTED_EDGE('',*,*,#9165,.F.);
#12177=ORIENTED_EDGE('',*,*,#9166,.F.);
#12178=ORIENTED_EDGE('',*,*,#9167,.F.);
#12179=ORIENTED_EDGE('',*,*,#9168,.T.);
#12180=ORIENTED_EDGE('',*,*,#9169,.T.);
#12181=ORIENTED_EDGE('',*,*,#9170,.T.);
#12182=ORIENTED_EDGE('',*,*,#9171,.F.);
#12183=ORIENTED_EDGE('',*,*,#9172,.T.);
#12184=ORIENTED_EDGE('',*,*,#9171,.T.);
#12185=ORIENTED_EDGE('',*,*,#9173,.T.);
#12186=ORIENTED_EDGE('',*,*,#9174,.F.);
#12187=ORIENTED_EDGE('',*,*,#9175,.T.);
#12188=ORIENTED_EDGE('',*,*,#9174,.T.);
#12189=ORIENTED_EDGE('',*,*,#9176,.T.);
#12190=ORIENTED_EDGE('',*,*,#9177,.F.);
#12191=ORIENTED_EDGE('',*,*,#9178,.T.);
#12192=ORIENTED_EDGE('',*,*,#9177,.T.);
#12193=ORIENTED_EDGE('',*,*,#9179,.T.);
#12194=ORIENTED_EDGE('',*,*,#9180,.F.);
#12195=ORIENTED_EDGE('',*,*,#9181,.T.);
#12196=ORIENTED_EDGE('',*,*,#9180,.T.);
#12197=ORIENTED_EDGE('',*,*,#9182,.T.);
#12198=ORIENTED_EDGE('',*,*,#9183,.F.);
#12199=ORIENTED_EDGE('',*,*,#9184,.T.);
#12200=ORIENTED_EDGE('',*,*,#9183,.T.);
#12201=ORIENTED_EDGE('',*,*,#9185,.T.);
#12202=ORIENTED_EDGE('',*,*,#9186,.F.);
#12203=ORIENTED_EDGE('',*,*,#9187,.T.);
#12204=ORIENTED_EDGE('',*,*,#9186,.T.);
#12205=ORIENTED_EDGE('',*,*,#9188,.T.);
#12206=ORIENTED_EDGE('',*,*,#9189,.F.);
#12207=ORIENTED_EDGE('',*,*,#9190,.T.);
#12208=ORIENTED_EDGE('',*,*,#9191,.T.);
#12209=ORIENTED_EDGE('',*,*,#9192,.T.);
#12210=ORIENTED_EDGE('',*,*,#9193,.F.);
#12211=ORIENTED_EDGE('',*,*,#9194,.T.);
#12212=ORIENTED_EDGE('',*,*,#9195,.T.);
#12213=ORIENTED_EDGE('',*,*,#9196,.T.);
#12214=ORIENTED_EDGE('',*,*,#9197,.F.);
#12215=ORIENTED_EDGE('',*,*,#9198,.T.);
#12216=ORIENTED_EDGE('',*,*,#9197,.T.);
#12217=ORIENTED_EDGE('',*,*,#9199,.T.);
#12218=ORIENTED_EDGE('',*,*,#9160,.T.);
#12219=ORIENTED_EDGE('',*,*,#9200,.F.);
#12220=ORIENTED_EDGE('',*,*,#9201,.T.);
#12221=ORIENTED_EDGE('',*,*,#9202,.T.);
#12222=ORIENTED_EDGE('',*,*,#9203,.T.);
#12223=ORIENTED_EDGE('',*,*,#9195,.F.);
#12224=ORIENTED_EDGE('',*,*,#9204,.F.);
#12225=ORIENTED_EDGE('',*,*,#9074,.T.);
#12226=ORIENTED_EDGE('',*,*,#9205,.T.);
#12227=ORIENTED_EDGE('',*,*,#9167,.T.);
#12228=ORIENTED_EDGE('',*,*,#9206,.F.);
#12229=ORIENTED_EDGE('',*,*,#9071,.T.);
#12230=ORIENTED_EDGE('',*,*,#9207,.T.);
#12231=ORIENTED_EDGE('',*,*,#9157,.T.);
#12232=ORIENTED_EDGE('',*,*,#9207,.F.);
#12233=ORIENTED_EDGE('',*,*,#9076,.T.);
#12234=ORIENTED_EDGE('',*,*,#9204,.T.);
#12235=ORIENTED_EDGE('',*,*,#9166,.T.);
#12236=ORIENTED_EDGE('',*,*,#9208,.F.);
#12237=ORIENTED_EDGE('',*,*,#9209,.T.);
#12238=ORIENTED_EDGE('',*,*,#9210,.F.);
#12239=ORIENTED_EDGE('',*,*,#9158,.T.);
#12240=ORIENTED_EDGE('',*,*,#9211,.F.);
#12241=ORIENTED_EDGE('',*,*,#9083,.T.);
#12242=ORIENTED_EDGE('',*,*,#9212,.T.);
#12243=ORIENTED_EDGE('',*,*,#9152,.T.);
#12244=ORIENTED_EDGE('',*,*,#9213,.F.);
#12245=ORIENTED_EDGE('',*,*,#9212,.F.);
#12246=ORIENTED_EDGE('',*,*,#9079,.T.);
#12247=ORIENTED_EDGE('',*,*,#9214,.T.);
#12248=ORIENTED_EDGE('',*,*,#9153,.T.);
#12249=ORIENTED_EDGE('',*,*,#9214,.F.);
#12250=ORIENTED_EDGE('',*,*,#9084,.T.);
#12251=ORIENTED_EDGE('',*,*,#9215,.T.);
#12252=ORIENTED_EDGE('',*,*,#9216,.F.);
#12253=ORIENTED_EDGE('',*,*,#9154,.T.);
#12254=ORIENTED_EDGE('',*,*,#9215,.F.);
#12255=ORIENTED_EDGE('',*,*,#9082,.T.);
#12256=ORIENTED_EDGE('',*,*,#9211,.T.);
#12257=ORIENTED_EDGE('',*,*,#9217,.T.);
#12258=ORIENTED_EDGE('',*,*,#9200,.T.);
#12259=ORIENTED_EDGE('',*,*,#9163,.T.);
#12260=ORIENTED_EDGE('',*,*,#9218,.F.);
#12261=ORIENTED_EDGE('',*,*,#9219,.F.);
#12262=ORIENTED_EDGE('',*,*,#9220,.F.);
#12263=ORIENTED_EDGE('',*,*,#9221,.F.);
#12264=ORIENTED_EDGE('',*,*,#9222,.F.);
#12265=ORIENTED_EDGE('',*,*,#9223,.F.);
#12266=ORIENTED_EDGE('',*,*,#9224,.F.);
#12267=ORIENTED_EDGE('',*,*,#9225,.F.);
#12268=ORIENTED_EDGE('',*,*,#9226,.F.);
#12269=ORIENTED_EDGE('',*,*,#9227,.F.);
#12270=ORIENTED_EDGE('',*,*,#9228,.F.);
#12271=ORIENTED_EDGE('',*,*,#9229,.F.);
#12272=ORIENTED_EDGE('',*,*,#9230,.F.);
#12273=ORIENTED_EDGE('',*,*,#9231,.F.);
#12274=ORIENTED_EDGE('',*,*,#9232,.F.);
#12275=ORIENTED_EDGE('',*,*,#9233,.F.);
#12276=ORIENTED_EDGE('',*,*,#9234,.F.);
#12277=ORIENTED_EDGE('',*,*,#9235,.F.);
#12278=ORIENTED_EDGE('',*,*,#9236,.F.);
#12279=ORIENTED_EDGE('',*,*,#9086,.T.);
#12280=ORIENTED_EDGE('',*,*,#9237,.F.);
#12281=ORIENTED_EDGE('',*,*,#9109,.T.);
#12282=ORIENTED_EDGE('',*,*,#9238,.F.);
#12283=ORIENTED_EDGE('',*,*,#9239,.F.);
#12284=ORIENTED_EDGE('',*,*,#9240,.T.);
#12285=ORIENTED_EDGE('',*,*,#9229,.T.);
#12286=ORIENTED_EDGE('',*,*,#9241,.F.);
#12287=ORIENTED_EDGE('',*,*,#9227,.T.);
#12288=ORIENTED_EDGE('',*,*,#9099,.T.);
#12289=ORIENTED_EDGE('',*,*,#9233,.T.);
#12290=ORIENTED_EDGE('',*,*,#9096,.F.);
#12291=ORIENTED_EDGE('',*,*,#9231,.T.);
#12292=ORIENTED_EDGE('',*,*,#9242,.F.);
#12293=ORIENTED_EDGE('',*,*,#9235,.T.);
#12294=ORIENTED_EDGE('',*,*,#9243,.T.);
#12295=ORIENTED_EDGE('',*,*,#9221,.T.);
#12296=ORIENTED_EDGE('',*,*,#9095,.T.);
#12297=ORIENTED_EDGE('',*,*,#9104,.T.);
#12298=ORIENTED_EDGE('',*,*,#9244,.T.);
#12299=ORIENTED_EDGE('',*,*,#9224,.T.);
#12300=ORIENTED_EDGE('',*,*,#9241,.T.);
#12301=ORIENTED_EDGE('',*,*,#9228,.T.);
#12302=ORIENTED_EDGE('',*,*,#9098,.T.);
#12303=ORIENTED_EDGE('',*,*,#9092,.T.);
#12304=ORIENTED_EDGE('',*,*,#9236,.T.);
#12305=ORIENTED_EDGE('',*,*,#9222,.T.);
#12306=ORIENTED_EDGE('',*,*,#9243,.F.);
#12307=ORIENTED_EDGE('',*,*,#9234,.T.);
#12308=ORIENTED_EDGE('',*,*,#9245,.T.);
#12309=ORIENTED_EDGE('',*,*,#9108,.T.);
#12310=ORIENTED_EDGE('',*,*,#9246,.T.);
#12311=ORIENTED_EDGE('',*,*,#9247,.T.);
#12312=ORIENTED_EDGE('',*,*,#9088,.T.);
#12313=ORIENTED_EDGE('',*,*,#9248,.T.);
#12314=ORIENTED_EDGE('',*,*,#9249,.T.);
#12315=ORIENTED_EDGE('',*,*,#9250,.T.);
#12316=ORIENTED_EDGE('',*,*,#9251,.T.);
#12317=ORIENTED_EDGE('',*,*,#9252,.F.);
#12318=ORIENTED_EDGE('',*,*,#9253,.T.);
#12319=ORIENTED_EDGE('',*,*,#9254,.T.);
#12320=ORIENTED_EDGE('',*,*,#9191,.F.);
#12321=ORIENTED_EDGE('',*,*,#9255,.T.);
#12322=ORIENTED_EDGE('',*,*,#9256,.T.);
#12323=ORIENTED_EDGE('',*,*,#9252,.T.);
#12324=ORIENTED_EDGE('',*,*,#9257,.T.);
#12325=ORIENTED_EDGE('',*,*,#9112,.T.);
#12326=ORIENTED_EDGE('',*,*,#9258,.T.);
#12327=ORIENTED_EDGE('',*,*,#9193,.T.);
#12328=ORIENTED_EDGE('',*,*,#9259,.T.);
#12329=ORIENTED_EDGE('',*,*,#9260,.T.);
#12330=ORIENTED_EDGE('',*,*,#9250,.F.);
#12331=ORIENTED_EDGE('',*,*,#9261,.T.);
#12332=ORIENTED_EDGE('',*,*,#9262,.T.);
#12333=ORIENTED_EDGE('',*,*,#9263,.T.);
#12334=ORIENTED_EDGE('',*,*,#9264,.F.);
#12335=ORIENTED_EDGE('',*,*,#9265,.T.);
#12336=ORIENTED_EDGE('',*,*,#9266,.T.);
#12337=ORIENTED_EDGE('',*,*,#9169,.F.);
#12338=ORIENTED_EDGE('',*,*,#9267,.T.);
#12339=ORIENTED_EDGE('',*,*,#9268,.T.);
#12340=ORIENTED_EDGE('',*,*,#9264,.T.);
#12341=ORIENTED_EDGE('',*,*,#9269,.F.);
#12342=ORIENTED_EDGE('',*,*,#9150,.T.);
#12343=ORIENTED_EDGE('',*,*,#9270,.T.);
#12344=ORIENTED_EDGE('',*,*,#9271,.T.);
#12345=ORIENTED_EDGE('',*,*,#9262,.F.);
#12346=ORIENTED_EDGE('',*,*,#9272,.T.);
#12347=ORIENTED_EDGE('',*,*,#9273,.T.);
#12348=ORIENTED_EDGE('',*,*,#9274,.T.);
#12349=ORIENTED_EDGE('',*,*,#9275,.F.);
#12350=ORIENTED_EDGE('',*,*,#9276,.F.);
#12351=ORIENTED_EDGE('',*,*,#9277,.T.);
#12352=ORIENTED_EDGE('',*,*,#9278,.T.);
#12353=ORIENTED_EDGE('',*,*,#9273,.F.);
#12354=ORIENTED_EDGE('',*,*,#9279,.F.);
#12355=ORIENTED_EDGE('',*,*,#9280,.T.);
#12356=ORIENTED_EDGE('',*,*,#9281,.T.);
#12357=ORIENTED_EDGE('',*,*,#9277,.F.);
#12358=ORIENTED_EDGE('',*,*,#9282,.F.);
#12359=ORIENTED_EDGE('',*,*,#9275,.T.);
#12360=ORIENTED_EDGE('',*,*,#9283,.T.);
#12361=ORIENTED_EDGE('',*,*,#9280,.F.);
#12362=ORIENTED_EDGE('',*,*,#9284,.F.);
#12363=ORIENTED_EDGE('',*,*,#9285,.T.);
#12364=ORIENTED_EDGE('',*,*,#9286,.T.);
#12365=ORIENTED_EDGE('',*,*,#9287,.F.);
#12366=ORIENTED_EDGE('',*,*,#9288,.F.);
#12367=ORIENTED_EDGE('',*,*,#9289,.T.);
#12368=ORIENTED_EDGE('',*,*,#9290,.T.);
#12369=ORIENTED_EDGE('',*,*,#9285,.F.);
#12370=ORIENTED_EDGE('',*,*,#9291,.F.);
#12371=ORIENTED_EDGE('',*,*,#9292,.T.);
#12372=ORIENTED_EDGE('',*,*,#9293,.T.);
#12373=ORIENTED_EDGE('',*,*,#9289,.F.);
#12374=ORIENTED_EDGE('',*,*,#9294,.F.);
#12375=ORIENTED_EDGE('',*,*,#9287,.T.);
#12376=ORIENTED_EDGE('',*,*,#9295,.T.);
#12377=ORIENTED_EDGE('',*,*,#9292,.F.);
#12378=ORIENTED_EDGE('',*,*,#9296,.F.);
#12379=ORIENTED_EDGE('',*,*,#9297,.T.);
#12380=ORIENTED_EDGE('',*,*,#9298,.T.);
#12381=ORIENTED_EDGE('',*,*,#9299,.F.);
#12382=ORIENTED_EDGE('',*,*,#9300,.F.);
#12383=ORIENTED_EDGE('',*,*,#9301,.F.);
#12384=ORIENTED_EDGE('',*,*,#9218,.T.);
#12385=ORIENTED_EDGE('',*,*,#9162,.T.);
#12386=ORIENTED_EDGE('',*,*,#9302,.T.);
#12387=ORIENTED_EDGE('',*,*,#9301,.T.);
#12388=ORIENTED_EDGE('',*,*,#9303,.T.);
#12389=ORIENTED_EDGE('',*,*,#9304,.T.);
#12390=ORIENTED_EDGE('',*,*,#9305,.F.);
#12391=ORIENTED_EDGE('',*,*,#9304,.F.);
#12392=ORIENTED_EDGE('',*,*,#9306,.T.);
#12393=ORIENTED_EDGE('',*,*,#9300,.T.);
#12394=ORIENTED_EDGE('',*,*,#9307,.F.);
#12395=ORIENTED_EDGE('',*,*,#9308,.T.);
#12396=ORIENTED_EDGE('',*,*,#9309,.T.);
#12397=ORIENTED_EDGE('',*,*,#9296,.T.);
#12398=ORIENTED_EDGE('',*,*,#9294,.T.);
#12399=ORIENTED_EDGE('',*,*,#9291,.T.);
#12400=ORIENTED_EDGE('',*,*,#9288,.T.);
#12401=ORIENTED_EDGE('',*,*,#9284,.T.);
#12402=ORIENTED_EDGE('',*,*,#9282,.T.);
#12403=ORIENTED_EDGE('',*,*,#9279,.T.);
#12404=ORIENTED_EDGE('',*,*,#9276,.T.);
#12405=ORIENTED_EDGE('',*,*,#9257,.F.);
#12406=ORIENTED_EDGE('',*,*,#9249,.F.);
#12407=ORIENTED_EDGE('',*,*,#9256,.F.);
#12408=ORIENTED_EDGE('',*,*,#9310,.T.);
#12409=ORIENTED_EDGE('',*,*,#9272,.F.);
#12410=ORIENTED_EDGE('',*,*,#9261,.F.);
#12411=ORIENTED_EDGE('',*,*,#9268,.F.);
#12412=ORIENTED_EDGE('',*,*,#9311,.T.);
#12413=ORIENTED_EDGE('',*,*,#9306,.F.);
#12414=ORIENTED_EDGE('',*,*,#9303,.F.);
#12415=ORIENTED_EDGE('',*,*,#9309,.F.);
#12416=ORIENTED_EDGE('',*,*,#9312,.T.);
#12417=ORIENTED_EDGE('',*,*,#9110,.T.);
#12418=ORIENTED_EDGE('',*,*,#9258,.F.);
#12419=ORIENTED_EDGE('',*,*,#9111,.T.);
#12420=ORIENTED_EDGE('',*,*,#9237,.T.);
#12421=ORIENTED_EDGE('',*,*,#9313,.T.);
#12422=ORIENTED_EDGE('',*,*,#9314,.T.);
#12423=ORIENTED_EDGE('',*,*,#9159,.T.);
#12424=ORIENTED_EDGE('',*,*,#9210,.T.);
#12425=ORIENTED_EDGE('',*,*,#9315,.F.);
#12426=ORIENTED_EDGE('',*,*,#9201,.F.);
#12427=ORIENTED_EDGE('',*,*,#9194,.F.);
#12428=ORIENTED_EDGE('',*,*,#9198,.F.);
#12429=ORIENTED_EDGE('',*,*,#9217,.F.);
#12430=ORIENTED_EDGE('',*,*,#9213,.T.);
#12431=ORIENTED_EDGE('',*,*,#9155,.T.);
#12432=ORIENTED_EDGE('',*,*,#9216,.T.);
#12433=ORIENTED_EDGE('',*,*,#9219,.T.);
#12434=ORIENTED_EDGE('',*,*,#9305,.T.);
#12435=ORIENTED_EDGE('',*,*,#9311,.F.);
#12436=ORIENTED_EDGE('',*,*,#9267,.F.);
#12437=ORIENTED_EDGE('',*,*,#9168,.F.);
#12438=ORIENTED_EDGE('',*,*,#9172,.F.);
#12439=ORIENTED_EDGE('',*,*,#9175,.F.);
#12440=ORIENTED_EDGE('',*,*,#9178,.F.);
#12441=ORIENTED_EDGE('',*,*,#9181,.F.);
#12442=ORIENTED_EDGE('',*,*,#9184,.F.);
#12443=ORIENTED_EDGE('',*,*,#9187,.F.);
#12444=ORIENTED_EDGE('',*,*,#9316,.F.);
#12445=ORIENTED_EDGE('',*,*,#9144,.T.);
#12446=ORIENTED_EDGE('',*,*,#9136,.T.);
#12447=ORIENTED_EDGE('',*,*,#9151,.T.);
#12448=ORIENTED_EDGE('',*,*,#9269,.T.);
#12449=ORIENTED_EDGE('',*,*,#9310,.F.);
#12450=ORIENTED_EDGE('',*,*,#9255,.F.);
#12451=ORIENTED_EDGE('',*,*,#9190,.F.);
#12452=ORIENTED_EDGE('',*,*,#9205,.F.);
#12453=ORIENTED_EDGE('',*,*,#9075,.T.);
#12454=ORIENTED_EDGE('',*,*,#9206,.T.);
#12455=ORIENTED_EDGE('',*,*,#9156,.T.);
#12456=ORIENTED_EDGE('',*,*,#9314,.F.);
#12457=ORIENTED_EDGE('',*,*,#9317,.T.);
#12458=ORIENTED_EDGE('',*,*,#9318,.T.);
#12459=ORIENTED_EDGE('',*,*,#9164,.T.);
#12460=ORIENTED_EDGE('',*,*,#9270,.F.);
#12461=ORIENTED_EDGE('',*,*,#9149,.T.);
#12462=ORIENTED_EDGE('',*,*,#9140,.T.);
#12463=ORIENTED_EDGE('',*,*,#9146,.T.);
#12464=ORIENTED_EDGE('',*,*,#9319,.F.);
#12465=ORIENTED_EDGE('',*,*,#9188,.F.);
#12466=ORIENTED_EDGE('',*,*,#9185,.F.);
#12467=ORIENTED_EDGE('',*,*,#9182,.F.);
#12468=ORIENTED_EDGE('',*,*,#9179,.F.);
#12469=ORIENTED_EDGE('',*,*,#9176,.F.);
#12470=ORIENTED_EDGE('',*,*,#9173,.F.);
#12471=ORIENTED_EDGE('',*,*,#9170,.F.);
#12472=ORIENTED_EDGE('',*,*,#9266,.F.);
#12473=ORIENTED_EDGE('',*,*,#9320,.T.);
#12474=ORIENTED_EDGE('',*,*,#9302,.F.);
#12475=ORIENTED_EDGE('',*,*,#9161,.T.);
#12476=ORIENTED_EDGE('',*,*,#9199,.F.);
#12477=ORIENTED_EDGE('',*,*,#9196,.F.);
#12478=ORIENTED_EDGE('',*,*,#9203,.F.);
#12479=ORIENTED_EDGE('',*,*,#9321,.F.);
#12480=ORIENTED_EDGE('',*,*,#9208,.T.);
#12481=ORIENTED_EDGE('',*,*,#9165,.T.);
#12482=ORIENTED_EDGE('',*,*,#9318,.F.);
#12483=ORIENTED_EDGE('',*,*,#9322,.T.);
#12484=ORIENTED_EDGE('',*,*,#9248,.F.);
#12485=ORIENTED_EDGE('',*,*,#9091,.T.);
#12486=ORIENTED_EDGE('',*,*,#9323,.F.);
#12487=ORIENTED_EDGE('',*,*,#9223,.T.);
#12488=ORIENTED_EDGE('',*,*,#9239,.T.);
#12489=ORIENTED_EDGE('',*,*,#9225,.T.);
#12490=ORIENTED_EDGE('',*,*,#9244,.F.);
#12491=ORIENTED_EDGE('',*,*,#9103,.T.);
#12492=ORIENTED_EDGE('',*,*,#9245,.F.);
#12493=ORIENTED_EDGE('',*,*,#9324,.T.);
#12494=ORIENTED_EDGE('',*,*,#9259,.F.);
#12495=ORIENTED_EDGE('',*,*,#9192,.F.);
#12496=ORIENTED_EDGE('',*,*,#9254,.F.);
#12497=ORIENTED_EDGE('',*,*,#9325,.T.);
#12498=ORIENTED_EDGE('',*,*,#9265,.F.);
#12499=ORIENTED_EDGE('',*,*,#9326,.T.);
#12500=ORIENTED_EDGE('',*,*,#9297,.F.);
#12501=ORIENTED_EDGE('',*,*,#9320,.F.);
#12502=ORIENTED_EDGE('',*,*,#9298,.F.);
#12503=ORIENTED_EDGE('',*,*,#9326,.F.);
#12504=ORIENTED_EDGE('',*,*,#9263,.F.);
#12505=ORIENTED_EDGE('',*,*,#9327,.F.);
#12506=ORIENTED_EDGE('',*,*,#9251,.F.);
#12507=ORIENTED_EDGE('',*,*,#9328,.F.);
#12508=ORIENTED_EDGE('',*,*,#9329,.T.);
#12509=ORIENTED_EDGE('',*,*,#9330,.T.);
#12510=ORIENTED_EDGE('',*,*,#9295,.F.);
#12511=ORIENTED_EDGE('',*,*,#9286,.F.);
#12512=ORIENTED_EDGE('',*,*,#9290,.F.);
#12513=ORIENTED_EDGE('',*,*,#9293,.F.);
#12514=ORIENTED_EDGE('',*,*,#9283,.F.);
#12515=ORIENTED_EDGE('',*,*,#9274,.F.);
#12516=ORIENTED_EDGE('',*,*,#9278,.F.);
#12517=ORIENTED_EDGE('',*,*,#9281,.F.);
#12518=ORIENTED_EDGE('',*,*,#9299,.T.);
#12519=ORIENTED_EDGE('',*,*,#9330,.F.);
#12520=ORIENTED_EDGE('',*,*,#9331,.T.);
#12521=ORIENTED_EDGE('',*,*,#9307,.T.);
#12522=ORIENTED_EDGE('',*,*,#9253,.F.);
#12523=ORIENTED_EDGE('',*,*,#9327,.T.);
#12524=ORIENTED_EDGE('',*,*,#9271,.F.);
#12525=ORIENTED_EDGE('',*,*,#9325,.F.);
#12526=ORIENTED_EDGE('',*,*,#9260,.F.);
#12527=ORIENTED_EDGE('',*,*,#9324,.F.);
#12528=ORIENTED_EDGE('',*,*,#9332,.T.);
#12529=ORIENTED_EDGE('',*,*,#9328,.T.);
#12530=ORIENTED_EDGE('',*,*,#9246,.F.);
#12531=ORIENTED_EDGE('',*,*,#9107,.T.);
#12532=ORIENTED_EDGE('',*,*,#9312,.F.);
#12533=ORIENTED_EDGE('',*,*,#9308,.F.);
#12534=ORIENTED_EDGE('',*,*,#9331,.F.);
#12535=ORIENTED_EDGE('',*,*,#9329,.F.);
#12536=ORIENTED_EDGE('',*,*,#9332,.F.);
#12537=ORIENTED_EDGE('',*,*,#9247,.F.);
#12538=ORIENTED_EDGE('',*,*,#9322,.F.);
#12539=ORIENTED_EDGE('',*,*,#9317,.F.);
#12540=ORIENTED_EDGE('',*,*,#9313,.F.);
#12541=ORIENTED_EDGE('',*,*,#9085,.T.);
#12542=ORIENTED_EDGE('',*,*,#9202,.F.);
#12543=ORIENTED_EDGE('',*,*,#9315,.T.);
#12544=ORIENTED_EDGE('',*,*,#9209,.F.);
#12545=ORIENTED_EDGE('',*,*,#9321,.T.);
#12546=ORIENTED_EDGE('',*,*,#9319,.T.);
#12547=ORIENTED_EDGE('',*,*,#9145,.T.);
#12548=ORIENTED_EDGE('',*,*,#9316,.T.);
#12549=ORIENTED_EDGE('',*,*,#9189,.T.);
#12550=ORIENTED_EDGE('',*,*,#9238,.T.);
#12551=ORIENTED_EDGE('',*,*,#9105,.T.);
#12552=ORIENTED_EDGE('',*,*,#9100,.T.);
#12553=ORIENTED_EDGE('',*,*,#9230,.T.);
#12554=ORIENTED_EDGE('',*,*,#9240,.F.);
#12555=ORIENTED_EDGE('',*,*,#9226,.T.);
#12556=ORIENTED_EDGE('',*,*,#9323,.T.);
#12557=ORIENTED_EDGE('',*,*,#9090,.T.);
#12558=ORIENTED_EDGE('',*,*,#9097,.T.);
#12559=ORIENTED_EDGE('',*,*,#9232,.T.);
#12560=ORIENTED_EDGE('',*,*,#9242,.T.);
#12561=ORIENTED_EDGE('',*,*,#9220,.T.);
#16434=PLANE('',#18149);
#16435=PLANE('',#18151);
#16436=PLANE('',#18152);
#16437=PLANE('',#18153);
#16438=PLANE('',#18154);
#16439=PLANE('',#18156);
#16440=PLANE('',#18163);
#16441=PLANE('',#18164);
#16442=PLANE('',#18165);
#16443=PLANE('',#18166);
#16444=PLANE('',#18179);
#16445=PLANE('',#18180);
#16446=PLANE('',#18181);
#16447=PLANE('',#18182);
#16448=PLANE('',#18183);
#16449=PLANE('',#18184);
#16450=PLANE('',#18185);
#16451=PLANE('',#18186);
#16452=PLANE('',#18187);
#16453=PLANE('',#18188);
#16454=PLANE('',#18189);
#16455=PLANE('',#18190);
#16456=PLANE('',#18191);
#16457=PLANE('',#18192);
#16458=PLANE('',#18193);
#16459=PLANE('',#18194);
#16460=PLANE('',#18195);
#16461=PLANE('',#18196);
#16462=PLANE('',#18210);
#16463=PLANE('',#18211);
#16464=PLANE('',#18212);
#16465=PLANE('',#18213);
#16466=PLANE('',#18214);
#16467=PLANE('',#18215);
#16468=PLANE('',#18216);
#16469=PLANE('',#18217);
#16470=PLANE('',#18218);
#16471=PLANE('',#18221);
#16472=PLANE('',#18224);
#16473=PLANE('',#18225);
#16474=PLANE('',#18228);
#16475=PLANE('',#18234);
#16476=PLANE('',#18238);
#16477=PLANE('',#18242);
#16478=PLANE('',#18246);
#16479=PLANE('',#18247);
#16480=PLANE('',#18249);
#16481=PLANE('',#18250);
#16482=PLANE('',#18252);
#16483=PLANE('',#18255);
#16484=PLANE('',#18256);
#16485=PLANE('',#18257);
#16486=PLANE('',#18259);
#16487=PLANE('',#18260);
#16488=PLANE('',#18264);
#16489=PLANE('',#18265);
#16490=PLANE('',#18266);
#16491=PLANE('',#18267);
#16492=PLANE('',#18268);
#16493=PLANE('',#18269);
#16998=ADVANCED_FACE('',(#1663),#515,.T.);
#16999=ADVANCED_FACE('',(#1664),#516,.T.);
#17000=ADVANCED_FACE('',(#1665),#517,.T.);
#17001=ADVANCED_FACE('',(#1666),#518,.T.);
#17002=ADVANCED_FACE('',(#1667),#519,.T.);
#17003=ADVANCED_FACE('',(#1668),#520,.T.);
#17004=ADVANCED_FACE('',(#1669),#521,.T.);
#17005=ADVANCED_FACE('',(#1670),#522,.T.);
#17006=ADVANCED_FACE('',(#1671),#523,.T.);
#17007=ADVANCED_FACE('',(#1672),#407,.F.);
#17008=ADVANCED_FACE('',(#1673),#524,.T.);
#17009=ADVANCED_FACE('',(#1674),#385,.T.);
#17010=ADVANCED_FACE('',(#1675),#525,.T.);
#17011=ADVANCED_FACE('',(#1676),#386,.T.);
#17012=ADVANCED_FACE('',(#1677),#526,.T.);
#17013=ADVANCED_FACE('',(#1678),#408,.F.);
#17014=ADVANCED_FACE('',(#1679),#527,.T.);
#17015=ADVANCED_FACE('',(#1680),#16434,.F.);
#17016=ADVANCED_FACE('',(#1681),#16435,.F.);
#17017=ADVANCED_FACE('',(#1682),#16436,.F.);
#17018=ADVANCED_FACE('',(#1683),#16437,.F.);
#17019=ADVANCED_FACE('',(#1684),#16438,.F.);
#17020=ADVANCED_FACE('',(#1685),#16439,.F.);
#17021=ADVANCED_FACE('',(#1686),#528,.T.);
#17022=ADVANCED_FACE('',(#1687),#529,.F.);
#17023=ADVANCED_FACE('',(#1688),#16440,.T.);
#17024=ADVANCED_FACE('',(#1689,#880),#16441,.T.);
#17025=ADVANCED_FACE('',(#1690),#16442,.T.);
#17026=ADVANCED_FACE('',(#1691),#16443,.T.);
#17027=ADVANCED_FACE('',(#1692),#530,.T.);
#17028=ADVANCED_FACE('',(#1693),#531,.T.);
#17029=ADVANCED_FACE('',(#1694),#532,.F.);
#17030=ADVANCED_FACE('',(#1695),#533,.F.);
#17031=ADVANCED_FACE('',(#1696),#16444,.F.);
#17032=ADVANCED_FACE('',(#1697),#16445,.F.);
#17033=ADVANCED_FACE('',(#1698),#16446,.F.);
#17034=ADVANCED_FACE('',(#1699),#16447,.F.);
#17035=ADVANCED_FACE('',(#1700),#16448,.F.);
#17036=ADVANCED_FACE('',(#1701),#16449,.F.);
#17037=ADVANCED_FACE('',(#1702),#16450,.F.);
#17038=ADVANCED_FACE('',(#1703),#16451,.F.);
#17039=ADVANCED_FACE('',(#1704),#16452,.F.);
#17040=ADVANCED_FACE('',(#1705),#16453,.F.);
#17041=ADVANCED_FACE('',(#1706),#16454,.F.);
#17042=ADVANCED_FACE('',(#1707),#16455,.T.);
#17043=ADVANCED_FACE('',(#1708),#16456,.T.);
#17044=ADVANCED_FACE('',(#1709),#16457,.T.);
#17045=ADVANCED_FACE('',(#1710),#16458,.T.);
#17046=ADVANCED_FACE('',(#1711),#16459,.T.);
#17047=ADVANCED_FACE('',(#1712),#16460,.T.);
#17048=ADVANCED_FACE('',(#1713),#16461,.T.);
#17049=ADVANCED_FACE('',(#1714),#534,.F.);
#17050=ADVANCED_FACE('',(#1715),#535,.F.);
#17051=ADVANCED_FACE('',(#1716),#536,.F.);
#17052=ADVANCED_FACE('',(#1717),#537,.F.);
#17053=ADVANCED_FACE('',(#1718),#538,.T.);
#17054=ADVANCED_FACE('',(#1719),#16462,.F.);
#17055=ADVANCED_FACE('',(#1720),#16463,.F.);
#17056=ADVANCED_FACE('',(#1721),#16464,.F.);
#17057=ADVANCED_FACE('',(#1722),#16465,.F.);
#17058=ADVANCED_FACE('',(#1723),#16466,.T.);
#17059=ADVANCED_FACE('',(#1724),#16467,.F.);
#17060=ADVANCED_FACE('',(#1725),#16468,.F.);
#17061=ADVANCED_FACE('',(#1726),#16469,.F.);
#17062=ADVANCED_FACE('',(#1727),#16470,.F.);
#17063=ADVANCED_FACE('',(#1728),#16471,.F.);
#17064=ADVANCED_FACE('',(#1729),#16472,.F.);
#17065=ADVANCED_FACE('',(#1730),#16473,.F.);
#17066=ADVANCED_FACE('',(#1731),#16474,.F.);
#17067=ADVANCED_FACE('',(#1732),#539,.F.);
#17068=ADVANCED_FACE('',(#1733),#16475,.F.);
#17069=ADVANCED_FACE('',(#1734),#540,.F.);
#17070=ADVANCED_FACE('',(#1735),#16476,.F.);
#17071=ADVANCED_FACE('',(#1736),#541,.F.);
#17072=ADVANCED_FACE('',(#1737),#16477,.F.);
#17073=ADVANCED_FACE('',(#1738),#542,.F.);
#17074=ADVANCED_FACE('',(#1739),#16478,.F.);
#17075=ADVANCED_FACE('',(#1740),#16479,.F.);
#17076=ADVANCED_FACE('',(#1741),#16480,.F.);
#17077=ADVANCED_FACE('',(#1742),#16481,.T.);
#17078=ADVANCED_FACE('',(#1743,#881,#882),#16482,.T.);
#17079=ADVANCED_FACE('',(#1744),#543,.F.);
#17080=ADVANCED_FACE('',(#1745),#16483,.T.);
#17081=ADVANCED_FACE('',(#1746),#16484,.T.);
#17082=ADVANCED_FACE('',(#1747),#16485,.T.);
#17083=ADVANCED_FACE('',(#1748),#544,.T.);
#17084=ADVANCED_FACE('',(#1749,#883,#884),#16486,.T.);
#17085=ADVANCED_FACE('',(#1750),#16487,.T.);
#17086=ADVANCED_FACE('',(#1751),#545,.T.);
#17087=ADVANCED_FACE('',(#1752),#546,.T.);
#17088=ADVANCED_FACE('',(#1753),#16488,.F.);
#17089=ADVANCED_FACE('',(#1754),#16489,.F.);
#17090=ADVANCED_FACE('',(#1755),#16490,.T.);
#17091=ADVANCED_FACE('',(#1756),#16491,.F.);
#17092=ADVANCED_FACE('',(#1757),#16492,.T.);
#17093=ADVANCED_FACE('',(#1758),#16493,.F.);
#17794=CLOSED_SHELL('',(#16998,#16999,#17000,#17001,#17002,#17003,#17004,
#17005,#17006,#17007,#17008,#17009,#17010,#17011,#17012,#17013,#17014,#17015,
#17016,#17017,#17018,#17019,#17020,#17021,#17022,#17023,#17024,#17025,#17026,
#17027,#17028,#17029,#17030,#17031,#17032,#17033,#17034,#17035,#17036,#17037,
#17038,#17039,#17040,#17041,#17042,#17043,#17044,#17045,#17046,#17047,#17048,
#17049,#17050,#17051,#17052,#17053,#17054,#17055,#17056,#17057,#17058,#17059,
#17060,#17061,#17062,#17063,#17064,#17065,#17066,#17067,#17068,#17069,#17070,
#17071,#17072,#17073,#17074,#17075,#17076,#17077,#17078,#17079,#17080,#17081,
#17082,#17083,#17084,#17085,#17086,#17087,#17088,#17089,#17090,#17091,#17092,
#17093));
#18105=AXIS2_PLACEMENT_3D('',#25002,#20168,#20169);
#18106=AXIS2_PLACEMENT_3D('',#25003,#20170,#20171);
#18107=AXIS2_PLACEMENT_3D('',#25006,#20172,#20173);
#18108=AXIS2_PLACEMENT_3D('',#25008,#20174,#20175);
#18109=AXIS2_PLACEMENT_3D('',#25012,#20177,#20178);
#18110=AXIS2_PLACEMENT_3D('',#25014,#20179,#20180);
#18111=AXIS2_PLACEMENT_3D('',#25016,#20182,#20183);
#18112=AXIS2_PLACEMENT_3D('',#25018,#20185,#20186);
#18113=AXIS2_PLACEMENT_3D('',#25020,#20188,#20189);
#18114=AXIS2_PLACEMENT_3D('',#25023,#20190,#20191);
#18115=AXIS2_PLACEMENT_3D('',#25025,#20192,#20193);
#18116=AXIS2_PLACEMENT_3D('',#25029,#20195,#20196);
#18117=AXIS2_PLACEMENT_3D('',#25031,#20197,#20198);
#18118=AXIS2_PLACEMENT_3D('',#25033,#20200,#20201);
#18119=AXIS2_PLACEMENT_3D('',#25035,#20203,#20204);
#18120=AXIS2_PLACEMENT_3D('',#25037,#20206,#20207);
#18121=AXIS2_PLACEMENT_3D('',#25040,#20208,#20209);
#18122=AXIS2_PLACEMENT_3D('',#25042,#20210,#20211);
#18123=AXIS2_PLACEMENT_3D('',#25046,#20213,#20214);
#18124=AXIS2_PLACEMENT_3D('',#25048,#20215,#20216);
#18125=AXIS2_PLACEMENT_3D('',#25050,#20218,#20219);
#18126=AXIS2_PLACEMENT_3D('',#25052,#20221,#20222);
#18127=AXIS2_PLACEMENT_3D('',#25065,#20224,#20225);
#18128=AXIS2_PLACEMENT_3D('',#25067,#20226,#20227);
#18129=AXIS2_PLACEMENT_3D('',#25069,#20228,#20229);
#18130=AXIS2_PLACEMENT_3D('',#25070,#20230,#20231);
#18131=AXIS2_PLACEMENT_3D('',#25071,#20232,#20233);
#18132=AXIS2_PLACEMENT_3D('',#25074,#20234,#20235);
#18133=AXIS2_PLACEMENT_3D('',#25077,#20237,#20238);
#18134=AXIS2_PLACEMENT_3D('',#25079,#20240,#20241);
#18135=AXIS2_PLACEMENT_3D('',#25080,#20242,#20243);
#18136=AXIS2_PLACEMENT_3D('',#25081,#20244,#20245);
#18137=AXIS2_PLACEMENT_3D('',#25084,#20246,#20247);
#18138=AXIS2_PLACEMENT_3D('',#25095,#20254,#20255);
#18139=AXIS2_PLACEMENT_3D('',#25096,#20256,#20257);
#18140=AXIS2_PLACEMENT_3D('',#25097,#20258,#20259);
#18141=AXIS2_PLACEMENT_3D('',#25100,#20260,#20261);
#18142=AXIS2_PLACEMENT_3D('',#25102,#20262,#20263);
#18143=AXIS2_PLACEMENT_3D('',#25116,#20266,#20267);
#18144=AXIS2_PLACEMENT_3D('',#25118,#20268,#20269);
#18145=AXIS2_PLACEMENT_3D('',#25119,#20270,#20271);
#18146=AXIS2_PLACEMENT_3D('',#25120,#20272,#20273);
#18147=AXIS2_PLACEMENT_3D('',#25121,#20274,#20275);
#18148=AXIS2_PLACEMENT_3D('',#25126,#20278,#20279);
#18149=AXIS2_PLACEMENT_3D('',#25127,#20280,#20281);
#18150=AXIS2_PLACEMENT_3D('',#25132,#20283,#20284);
#18151=AXIS2_PLACEMENT_3D('',#25138,#20288,#20289);
#18152=AXIS2_PLACEMENT_3D('',#25144,#20293,#20294);
#18153=AXIS2_PLACEMENT_3D('',#25150,#20298,#20299);
#18154=AXIS2_PLACEMENT_3D('',#25156,#20303,#20304);
#18155=AXIS2_PLACEMENT_3D('',#25163,#20308,#20309);
#18156=AXIS2_PLACEMENT_3D('',#25164,#20310,#20311);
#18157=AXIS2_PLACEMENT_3D('',#25167,#20314,#20315);
#18158=AXIS2_PLACEMENT_3D('',#25170,#20316,#20317);
#18159=AXIS2_PLACEMENT_3D('',#25174,#20319,#20320);
#18160=AXIS2_PLACEMENT_3D('',#25176,#20322,#20323);
#18161=AXIS2_PLACEMENT_3D('',#25182,#20326,#20327);
#18162=AXIS2_PLACEMENT_3D('',#25185,#20329,#20330);
#18163=AXIS2_PLACEMENT_3D('',#25186,#20331,#20332);
#18164=AXIS2_PLACEMENT_3D('',#25194,#20338,#20339);
#18165=AXIS2_PLACEMENT_3D('',#25196,#20341,#20342);
#18166=AXIS2_PLACEMENT_3D('',#25203,#20347,#20348);
#18167=AXIS2_PLACEMENT_3D('',#25204,#20349,#20350);
#18168=AXIS2_PLACEMENT_3D('',#25207,#20351,#20352);
#18169=AXIS2_PLACEMENT_3D('',#25211,#20354,#20355);
#18170=AXIS2_PLACEMENT_3D('',#25213,#20357,#20358);
#18171=AXIS2_PLACEMENT_3D('',#25216,#20359,#20360);
#18172=AXIS2_PLACEMENT_3D('',#25220,#20362,#20363);
#18173=AXIS2_PLACEMENT_3D('',#25222,#20365,#20366);
#18174=AXIS2_PLACEMENT_3D('',#25225,#20367,#20368);
#18175=AXIS2_PLACEMENT_3D('',#25229,#20370,#20371);
#18176=AXIS2_PLACEMENT_3D('',#25231,#20373,#20374);
#18177=AXIS2_PLACEMENT_3D('',#25234,#20375,#20376);
#18178=AXIS2_PLACEMENT_3D('',#25238,#20378,#20379);
#18179=AXIS2_PLACEMENT_3D('',#25240,#20381,#20382);
#18180=AXIS2_PLACEMENT_3D('',#25249,#20387,#20388);
#18181=AXIS2_PLACEMENT_3D('',#25255,#20392,#20393);
#18182=AXIS2_PLACEMENT_3D('',#25261,#20397,#20398);
#18183=AXIS2_PLACEMENT_3D('',#25267,#20402,#20403);
#18184=AXIS2_PLACEMENT_3D('',#25273,#20407,#20408);
#18185=AXIS2_PLACEMENT_3D('',#25279,#20412,#20413);
#18186=AXIS2_PLACEMENT_3D('',#25285,#20417,#20418);
#18187=AXIS2_PLACEMENT_3D('',#25294,#20423,#20424);
#18188=AXIS2_PLACEMENT_3D('',#25303,#20429,#20430);
#18189=AXIS2_PLACEMENT_3D('',#25308,#20434,#20435);
#18190=AXIS2_PLACEMENT_3D('',#25314,#20439,#20440);
#18191=AXIS2_PLACEMENT_3D('',#25317,#20443,#20444);
#18192=AXIS2_PLACEMENT_3D('',#25320,#20447,#20448);
#18193=AXIS2_PLACEMENT_3D('',#25326,#20452,#20453);
#18194=AXIS2_PLACEMENT_3D('',#25331,#20457,#20458);
#18195=AXIS2_PLACEMENT_3D('',#25333,#20460,#20461);
#18196=AXIS2_PLACEMENT_3D('',#25337,#20464,#20465);
#18197=AXIS2_PLACEMENT_3D('',#25342,#20469,#20470);
#18198=AXIS2_PLACEMENT_3D('',#25345,#20471,#20472);
#18199=AXIS2_PLACEMENT_3D('',#25349,#20474,#20475);
#18200=AXIS2_PLACEMENT_3D('',#25351,#20477,#20478);
#18201=AXIS2_PLACEMENT_3D('',#25354,#20479,#20480);
#18202=AXIS2_PLACEMENT_3D('',#25358,#20482,#20483);
#18203=AXIS2_PLACEMENT_3D('',#25360,#20485,#20486);
#18204=AXIS2_PLACEMENT_3D('',#25362,#20487,#20488);
#18205=AXIS2_PLACEMENT_3D('',#25365,#20490,#20491);
#18206=AXIS2_PLACEMENT_3D('',#25367,#20493,#20494);
#18207=AXIS2_PLACEMENT_3D('',#25369,#20495,#20496);
#18208=AXIS2_PLACEMENT_3D('',#25372,#20498,#20499);
#18209=AXIS2_PLACEMENT_3D('',#25374,#20501,#20502);
#18210=AXIS2_PLACEMENT_3D('',#25379,#20507,#20508);
#18211=AXIS2_PLACEMENT_3D('',#25382,#20511,#20512);
#18212=AXIS2_PLACEMENT_3D('',#25383,#20513,#20514);
#18213=AXIS2_PLACEMENT_3D('',#25386,#20517,#20518);
#18214=AXIS2_PLACEMENT_3D('',#25388,#20520,#20521);
#18215=AXIS2_PLACEMENT_3D('',#25389,#20522,#20523);
#18216=AXIS2_PLACEMENT_3D('',#25393,#20526,#20527);
#18217=AXIS2_PLACEMENT_3D('',#25397,#20530,#20531);
#18218=AXIS2_PLACEMENT_3D('',#25406,#20536,#20537);
#18219=AXIS2_PLACEMENT_3D('',#25408,#20538,#20539);
#18220=AXIS2_PLACEMENT_3D('',#25412,#20542,#20543);
#18221=AXIS2_PLACEMENT_3D('',#25413,#20544,#20545);
#18222=AXIS2_PLACEMENT_3D('',#25414,#20546,#20547);
#18223=AXIS2_PLACEMENT_3D('',#25418,#20550,#20551);
#18224=AXIS2_PLACEMENT_3D('',#25419,#20552,#20553);
#18225=AXIS2_PLACEMENT_3D('',#25428,#20558,#20559);
#18226=AXIS2_PLACEMENT_3D('',#25430,#20560,#20561);
#18227=AXIS2_PLACEMENT_3D('',#25434,#20564,#20565);
#18228=AXIS2_PLACEMENT_3D('',#25435,#20566,#20567);
#18229=AXIS2_PLACEMENT_3D('',#25440,#20570,#20571);
#18230=AXIS2_PLACEMENT_3D('',#25441,#20572,#20573);
#18231=AXIS2_PLACEMENT_3D('',#25442,#20574,#20575);
#18232=AXIS2_PLACEMENT_3D('',#25447,#20577,#20578);
#18233=AXIS2_PLACEMENT_3D('',#25450,#20580,#20581);
#18234=AXIS2_PLACEMENT_3D('',#25451,#20582,#20583);
#18235=AXIS2_PLACEMENT_3D('',#25457,#20587,#20588);
#18236=AXIS2_PLACEMENT_3D('',#25461,#20590,#20591);
#18237=AXIS2_PLACEMENT_3D('',#25462,#20592,#20593);
#18238=AXIS2_PLACEMENT_3D('',#25463,#20594,#20595);
#18239=AXIS2_PLACEMENT_3D('',#25466,#20598,#20599);
#18240=AXIS2_PLACEMENT_3D('',#25471,#20601,#20602);
#18241=AXIS2_PLACEMENT_3D('',#25474,#20604,#20605);
#18242=AXIS2_PLACEMENT_3D('',#25475,#20606,#20607);
#18243=AXIS2_PLACEMENT_3D('',#25481,#20611,#20612);
#18244=AXIS2_PLACEMENT_3D('',#25485,#20614,#20615);
#18245=AXIS2_PLACEMENT_3D('',#25486,#20616,#20617);
#18246=AXIS2_PLACEMENT_3D('',#25487,#20618,#20619);
#18247=AXIS2_PLACEMENT_3D('',#25490,#20622,#20623);
#18248=AXIS2_PLACEMENT_3D('',#25493,#20624,#20625);
#18249=AXIS2_PLACEMENT_3D('',#25501,#20630,#20631);
#18250=AXIS2_PLACEMENT_3D('',#25506,#20635,#20636);
#18251=AXIS2_PLACEMENT_3D('',#25509,#20638,#20639);
#18252=AXIS2_PLACEMENT_3D('',#25510,#20640,#20641);
#18253=AXIS2_PLACEMENT_3D('',#25516,#20645,#20646);
#18254=AXIS2_PLACEMENT_3D('',#25519,#20649,#20650);
#18255=AXIS2_PLACEMENT_3D('',#25520,#20651,#20652);
#18256=AXIS2_PLACEMENT_3D('',#25526,#20657,#20658);
#18257=AXIS2_PLACEMENT_3D('',#25530,#20661,#20662);
#18258=AXIS2_PLACEMENT_3D('',#25538,#20670,#20671);
#18259=AXIS2_PLACEMENT_3D('',#25540,#20673,#20674);
#18260=AXIS2_PLACEMENT_3D('',#25547,#20679,#20680);
#18261=AXIS2_PLACEMENT_3D('',#25549,#20682,#20683);
#18262=AXIS2_PLACEMENT_3D('',#25550,#20684,#20685);
#18263=AXIS2_PLACEMENT_3D('',#25551,#20686,#20687);
#18264=AXIS2_PLACEMENT_3D('',#25552,#20688,#20689);
#18265=AXIS2_PLACEMENT_3D('',#25553,#20690,#20691);
#18266=AXIS2_PLACEMENT_3D('',#25554,#20692,#20693);
#18267=AXIS2_PLACEMENT_3D('',#25555,#20694,#20695);
#18268=AXIS2_PLACEMENT_3D('',#25556,#20696,#20697);
#18269=AXIS2_PLACEMENT_3D('',#25557,#20698,#20699);
#20168=DIRECTION('axis',(0.,0.,1.));
#20169=DIRECTION('refdir',(1.,0.,0.));
#20170=DIRECTION('center_axis',(-2.E-15,0.,-1.));
#20171=DIRECTION('ref_axis',(0.,1.,0.));
#20172=DIRECTION('center_axis',(-0.707106781186422,-2.63949809299824E-13,
-0.707106781186673));
#20173=DIRECTION('ref_axis',(0.707106781186673,5.14283623687556E-12,-0.707106781186422));
#20174=DIRECTION('center_axis',(-0.707106781186407,2.94314808737385E-13,
0.707106781186688));
#20175=DIRECTION('ref_axis',(0.707106781186688,-1.95499137120663E-12,0.707106781186407));
#20176=DIRECTION('',(2.E-15,-2.492418787323E-17,1.));
#20177=DIRECTION('center_axis',(-0.707106781186639,-1.64750638840042E-13,
-0.707106781186456));
#20178=DIRECTION('ref_axis',(0.707106781186456,1.02903869399948E-12,-0.707106781186639));
#20179=DIRECTION('center_axis',(-0.707106781186606,1.10586045248791E-13,
0.707106781186489));
#20180=DIRECTION('ref_axis',(0.707106781186489,-2.4427646214065E-13,0.707106781186606));
#20181=DIRECTION('',(-2.E-15,2.492418787323E-17,-1.));
#20182=DIRECTION('center_axis',(1.,-1.E-15,-2.E-15));
#20183=DIRECTION('ref_axis',(-1.E-15,-1.,2.E-30));
#20184=DIRECTION('',(1.,-1.E-15,-2.E-15));
#20185=DIRECTION('center_axis',(-1.,1.E-15,2.E-15));
#20186=DIRECTION('ref_axis',(2.E-15,-2.E-30,1.));
#20187=DIRECTION('',(-1.,1.E-15,1.7831595655029E-15));
#20188=DIRECTION('center_axis',(-2.E-15,0.,-1.));
#20189=DIRECTION('ref_axis',(-1.,0.,2.E-15));
#20190=DIRECTION('center_axis',(-0.707106781186533,-3.78536648393456E-14,
-0.707106781186562));
#20191=DIRECTION('ref_axis',(0.707106781186562,2.12340059618623E-12,-0.707106781186533));
#20192=DIRECTION('center_axis',(-0.70710678118642,2.63436887012028E-13,
0.707106781186675));
#20193=DIRECTION('ref_axis',(0.707106781186675,4.53699827383031E-13,0.707106781186421));
#20194=DIRECTION('',(1.25746720174781E-15,7.42532798252193E-31,1.));
#20195=DIRECTION('center_axis',(-0.707106781186551,2.46202698142038E-15,
-0.707106781186544));
#20196=DIRECTION('ref_axis',(0.707106781186544,-5.81158480807406E-13,-0.707106781186551));
#20197=DIRECTION('center_axis',(-0.707106781186549,-6.5654052837888E-15,
0.707106781186546));
#20198=DIRECTION('ref_axis',(0.707106781186546,2.87235972405227E-13,0.707106781186549));
#20199=DIRECTION('',(-1.25746720174781E-15,-7.42532798252193E-31,-1.));
#20200=DIRECTION('center_axis',(1.,-1.E-15,-2.E-15));
#20201=DIRECTION('ref_axis',(-2.E-15,2.E-30,-1.));
#20202=DIRECTION('',(1.,-1.E-15,-2.E-15));
#20203=DIRECTION('center_axis',(-1.,1.E-15,2.E-15));
#20204=DIRECTION('ref_axis',(2.E-15,1.68404344971007E-31,1.));
#20205=DIRECTION('',(-1.,1.E-15,2.E-15));
#20206=DIRECTION('center_axis',(-2.E-15,0.,-1.));
#20207=DIRECTION('ref_axis',(8.67361737988403E-16,1.,-1.73472347597681E-30));
#20208=DIRECTION('center_axis',(-0.707106781186533,-3.88795094149376E-14,
-0.707106781186562));
#20209=DIRECTION('ref_axis',(0.707106781186562,1.8346264764677E-13,-0.707106781186533));
#20210=DIRECTION('center_axis',(-0.707106781186432,2.39739877315856E-13,
0.707106781186663));
#20211=DIRECTION('ref_axis',(0.707106781186663,-1.65337637937498E-12,0.707106781186432));
#20212=DIRECTION('',(2.E-15,-4.20505361484229E-17,1.));
#20213=DIRECTION('center_axis',(-0.707106781186573,-9.17105050579052E-14,
-0.707106781186522));
#20214=DIRECTION('ref_axis',(0.707106781186522,1.86047575754184E-12,-0.707106781186573));
#20215=DIRECTION('center_axis',(-0.707106781186607,1.60442091622566E-13,
0.707106781186488));
#20216=DIRECTION('ref_axis',(0.707106781186488,-1.11785938449787E-12,0.707106781186607));
#20217=DIRECTION('',(-2.E-15,4.20505361484229E-17,-1.));
#20218=DIRECTION('center_axis',(1.,-1.E-15,-2.E-15));
#20219=DIRECTION('ref_axis',(-2.E-15,-1.68404344971007E-31,-1.));
#20220=DIRECTION('',(1.,-1.E-15,-2.E-15));
#20221=DIRECTION('center_axis',(-1.,1.E-15,2.E-15));
#20222=DIRECTION('ref_axis',(2.E-15,1.68404344971007E-31,1.));
#20223=DIRECTION('',(-1.,1.E-15,2.E-15));
#20224=DIRECTION('center_axis',(1.,-1.E-15,-2.E-15));
#20225=DIRECTION('ref_axis',(-2.E-15,2.E-30,-1.));
#20226=DIRECTION('center_axis',(2.E-15,0.,1.));
#20227=DIRECTION('ref_axis',(1.,0.,-2.E-15));
#20228=DIRECTION('center_axis',(-1.E-15,-1.,0.));
#20229=DIRECTION('ref_axis',(-1.,1.E-15,0.));
#20230=DIRECTION('center_axis',(-2.E-15,0.,-1.));
#20231=DIRECTION('ref_axis',(1.,0.,-2.E-15));
#20232=DIRECTION('center_axis',(1.E-15,1.,0.));
#20233=DIRECTION('ref_axis',(1.,-1.E-15,0.));
#20234=DIRECTION('center_axis',(-1.E-15,-1.,0.));
#20235=DIRECTION('ref_axis',(-1.,1.E-15,0.));
#20236=DIRECTION('',(1.E-15,1.,0.));
#20237=DIRECTION('center_axis',(-1.E-15,-1.,-2.11758236813575E-19));
#20238=DIRECTION('ref_axis',(-2.11758236813575E-34,-2.11758236813575E-19,
1.));
#20239=DIRECTION('',(-1.E-15,-1.,0.));
#20240=DIRECTION('center_axis',(1.,0.,0.));
#20241=DIRECTION('ref_axis',(0.,0.,1.));
#20242=DIRECTION('center_axis',(-2.E-15,0.,-1.));
#20243=DIRECTION('ref_axis',(-1.,0.,2.E-15));
#20244=DIRECTION('center_axis',(-2.E-15,2.94543590196345E-19,-1.));
#20245=DIRECTION('ref_axis',(5.89087180392689E-34,1.,2.94543590196345E-19));
#20246=DIRECTION('center_axis',(-2.E-15,0.,-1.));
#20247=DIRECTION('ref_axis',(-1.,0.,2.E-15));
#20248=DIRECTION('',(2.E-15,-2.94543590196345E-19,1.));
#20249=DIRECTION('',(-2.E-15,0.,-1.));
#20250=DIRECTION('',(2.E-15,-2.94543590196345E-19,1.));
#20251=DIRECTION('',(-2.E-15,2.94543590196345E-19,-1.));
#20252=DIRECTION('',(-2.E-15,0.,-1.));
#20253=DIRECTION('',(-2.E-15,2.94543590196345E-19,-1.));
#20254=DIRECTION('center_axis',(1.,0.,0.));
#20255=DIRECTION('ref_axis',(0.,0.,1.));
#20256=DIRECTION('center_axis',(1.E-15,1.,0.));
#20257=DIRECTION('ref_axis',(1.,-1.E-15,0.));
#20258=DIRECTION('center_axis',(-1.E-15,-1.,0.));
#20259=DIRECTION('ref_axis',(-1.,1.E-15,0.));
#20260=DIRECTION('center_axis',(1.E-15,1.,0.));
#20261=DIRECTION('ref_axis',(1.,-1.E-15,0.));
#20262=DIRECTION('center_axis',(-1.E-15,-1.,-2.11758236813575E-19));
#20263=DIRECTION('ref_axis',(-2.11758236813575E-34,-2.11758236813575E-19,
1.));
#20264=DIRECTION('',(-1.E-15,-1.,0.));
#20265=DIRECTION('',(1.E-15,1.,0.));
#20266=DIRECTION('center_axis',(-1.,1.E-15,-1.46944695195361E-15));
#20267=DIRECTION('ref_axis',(-1.46944695195361E-15,1.46944695195362E-30,
1.));
#20268=DIRECTION('center_axis',(1.,-1.E-15,-2.E-15));
#20269=DIRECTION('ref_axis',(-2.E-15,2.E-30,-1.));
#20270=DIRECTION('center_axis',(2.E-15,0.,1.));
#20271=DIRECTION('ref_axis',(-1.,0.,2.E-15));
#20272=DIRECTION('center_axis',(-2.E-15,0.,-1.));
#20273=DIRECTION('ref_axis',(-1.,0.,2.E-15));
#20274=DIRECTION('center_axis',(-1.,1.E-15,2.E-15));
#20275=DIRECTION('ref_axis',(2.E-15,-2.E-30,1.));
#20276=DIRECTION('',(1.,-1.E-15,-2.E-15));
#20277=DIRECTION('',(-1.,1.E-15,2.E-15));
#20278=DIRECTION('center_axis',(1.,-1.E-15,-2.E-15));
#20279=DIRECTION('ref_axis',(1.E-15,1.,-2.E-30));
#20280=DIRECTION('center_axis',(-2.E-15,2.E-30,-1.));
#20281=DIRECTION('ref_axis',(1.E-15,1.,0.));
#20282=DIRECTION('',(-1.E-15,-1.,0.));
#20283=DIRECTION('center_axis',(2.E-15,0.,1.));
#20284=DIRECTION('ref_axis',(-1.,0.,2.E-15));
#20285=DIRECTION('',(1.,-1.E-15,-2.E-15));
#20286=DIRECTION('',(1.E-15,1.,0.));
#20287=DIRECTION('',(1.,-1.E-15,-2.E-15));
#20288=DIRECTION('center_axis',(1.E-15,1.,-3.67526160164598E-17));
#20289=DIRECTION('ref_axis',(-2.E-15,-3.67526160164578E-17,-1.));
#20290=DIRECTION('',(-2.E-15,-3.67526160164578E-17,-1.));
#20291=DIRECTION('',(2.E-15,3.67526160164578E-17,1.));
#20292=DIRECTION('',(1.,-1.E-15,-2.E-15));
#20293=DIRECTION('center_axis',(-2.E-15,2.E-30,-1.));
#20294=DIRECTION('ref_axis',(1.E-15,1.,0.));
#20295=DIRECTION('',(-1.E-15,-1.,0.));
#20296=DIRECTION('',(1.E-15,1.,0.));
#20297=DIRECTION('',(1.,-1.E-15,-2.E-15));
#20298=DIRECTION('center_axis',(1.E-15,1.,-2.E-30));
#20299=DIRECTION('ref_axis',(-2.E-15,1.44148758291472E-46,-1.));
#20300=DIRECTION('',(-2.E-15,0.,-1.));
#20301=DIRECTION('',(2.E-15,0.,1.));
#20302=DIRECTION('',(1.,-1.E-15,-2.E-15));
#20303=DIRECTION('center_axis',(2.E-15,0.,1.));
#20304=DIRECTION('ref_axis',(1.,-1.E-15,-2.E-15));
#20305=DIRECTION('',(1.E-15,1.,0.));
#20306=DIRECTION('',(-1.E-15,-1.,0.));
#20307=DIRECTION('',(1.,-1.E-15,-2.E-15));
#20308=DIRECTION('center_axis',(-2.E-15,0.,-1.));
#20309=DIRECTION('ref_axis',(1.,0.,-2.E-15));
#20310=DIRECTION('center_axis',(-1.E-15,-1.,1.23908819712631E-16));
#20311=DIRECTION('ref_axis',(2.E-15,1.23908819712629E-16,1.));
#20312=DIRECTION('',(-2.E-15,-1.23908819712629E-16,-1.));
#20313=DIRECTION('',(-2.E-15,2.11758236813575E-19,-1.));
#20314=DIRECTION('center_axis',(2.E-15,0.,1.));
#20315=DIRECTION('ref_axis',(0.,-1.,0.));
#20316=DIRECTION('center_axis',(-2.E-15,0.,-1.));
#20317=DIRECTION('ref_axis',(0.,1.,0.));
#20318=DIRECTION('',(-2.E-15,1.39036381887169E-17,-1.));
#20319=DIRECTION('center_axis',(2.E-15,-1.88507897725893E-17,1.));
#20320=DIRECTION('ref_axis',(1.,3.77015795451787E-32,-2.E-15));
#20321=DIRECTION('',(2.E-15,-1.39036381887169E-17,1.));
#20322=DIRECTION('center_axis',(-2.E-15,0.,-1.));
#20323=DIRECTION('ref_axis',(0.,1.,0.));
#20324=DIRECTION('',(2.E-15,-2.11758236813575E-19,1.));
#20325=DIRECTION('',(2.E-15,-2.11758236813575E-19,1.));
#20326=DIRECTION('center_axis',(2.E-15,0.,1.));
#20327=DIRECTION('ref_axis',(0.,1.,0.));
#20328=DIRECTION('',(-2.E-15,2.11758236813575E-19,-1.));
#20329=DIRECTION('center_axis',(-2.E-15,1.88507897725893E-17,-1.));
#20330=DIRECTION('ref_axis',(1.,3.77015795451787E-32,-2.E-15));
#20331=DIRECTION('center_axis',(-2.E-15,1.88507897725913E-17,-1.));
#20332=DIRECTION('ref_axis',(1.E-15,1.,1.88507897725894E-17));
#20333=DIRECTION('',(-1.E-15,-1.,-1.88507897725893E-17));
#20334=DIRECTION('',(-1.E-15,-1.,-1.88507897725893E-17));
#20335=DIRECTION('',(1.,-1.E-15,-2.E-15));
#20336=DIRECTION('',(-1.E-15,-1.,-1.88507897725893E-17));
#20337=DIRECTION('',(1.,-1.E-15,-2.E-15));
#20338=DIRECTION('center_axis',(1.,-1.E-15,-2.E-15));
#20339=DIRECTION('ref_axis',(-2.E-15,0.,-1.));
#20340=DIRECTION('',(-1.E-15,-1.,-1.88507897725893E-17));
#20341=DIRECTION('center_axis',(1.7831595655029E-15,-1.88507897725891E-17,
1.));
#20342=DIRECTION('ref_axis',(1.,-1.E-15,-1.7831595655029E-15));
#20343=DIRECTION('',(-1.E-15,-1.,-1.88507897725893E-17));
#20344=DIRECTION('',(-1.,1.E-15,1.7831595655029E-15));
#20345=DIRECTION('',(1.E-15,1.,1.88507897725893E-17));
#20346=DIRECTION('',(-1.,1.E-15,1.7831595655029E-15));
#20347=DIRECTION('center_axis',(-1.,1.E-15,2.E-15));
#20348=DIRECTION('ref_axis',(-1.E-15,-1.,1.44148758291472E-46));
#20349=DIRECTION('center_axis',(2.E-15,0.,1.));
#20350=DIRECTION('ref_axis',(-8.67361737988403E-16,-1.,1.73472347597681E-30));
#20351=DIRECTION('center_axis',(-2.E-15,0.,-1.));
#20352=DIRECTION('ref_axis',(8.67361737988403E-16,1.,-1.73472347597681E-30));
#20353=DIRECTION('',(-2.E-15,1.39036381887169E-17,-1.));
#20354=DIRECTION('center_axis',(2.E-15,0.,1.));
#20355=DIRECTION('ref_axis',(-8.67361737988403E-16,-1.,1.73472347597681E-30));
#20356=DIRECTION('',(2.E-15,-1.39036381887169E-17,1.));
#20357=DIRECTION('center_axis',(2.E-15,-1.39036381887169E-17,1.));
#20358=DIRECTION('ref_axis',(1.,2.78072763774338E-32,-2.E-15));
#20359=DIRECTION('center_axis',(-2.E-15,0.,-1.));
#20360=DIRECTION('ref_axis',(-1.,0.,2.E-15));
#20361=DIRECTION('',(-1.25746720174781E-15,1.39036381887162E-17,-1.));
#20362=DIRECTION('center_axis',(2.E-15,0.,1.));
#20363=DIRECTION('ref_axis',(-8.67361737988403E-16,-1.,1.73472347597681E-30));
#20364=DIRECTION('',(1.25746720174781E-15,-1.39036381887162E-17,1.));
#20365=DIRECTION('center_axis',(-2.E-15,0.,-1.));
#20366=DIRECTION('ref_axis',(1.0842021724855E-15,1.,-2.16840434497101E-30));
#20367=DIRECTION('center_axis',(2.E-15,-2.94543590196344E-19,1.));
#20368=DIRECTION('ref_axis',(1.,5.89087180392688E-34,-2.E-15));
#20369=DIRECTION('',(-2.E-15,2.11758236813575E-19,-1.));
#20370=DIRECTION('center_axis',(-2.E-15,0.,-1.));
#20371=DIRECTION('ref_axis',(1.0842021724855E-15,1.,-2.16840434497101E-30));
#20372=DIRECTION('',(2.E-15,-2.11758236813575E-19,1.));
#20373=DIRECTION('center_axis',(-2.E-15,2.11758236813575E-19,-1.));
#20374=DIRECTION('ref_axis',(-1.,-4.2351647362715E-34,2.E-15));
#20375=DIRECTION('center_axis',(2.E-15,0.,1.));
#20376=DIRECTION('ref_axis',(-1.,0.,2.E-15));
#20377=DIRECTION('',(-1.25746720174781E-15,2.11758236812832E-19,-1.));
#20378=DIRECTION('center_axis',(-2.E-15,0.,-1.));
#20379=DIRECTION('ref_axis',(-1.0842021724855E-15,-1.,2.16840434497101E-30));
#20380=DIRECTION('',(1.25746720174781E-15,-2.11758236812832E-19,1.));
#20381=DIRECTION('center_axis',(1.71087942067053E-15,-2.94543590196055E-19,
1.));
#20382=DIRECTION('ref_axis',(1.,-1.E-15,-1.71087942067053E-15));
#20383=DIRECTION('',(-1.,1.E-15,1.71087942067053E-15));
#20384=DIRECTION('',(1.E-15,1.,2.94543590196345E-19));
#20385=DIRECTION('',(1.,-1.E-15,-1.71087942067053E-15));
#20386=DIRECTION('',(1.E-15,1.,2.94543590196345E-19));
#20387=DIRECTION('center_axis',(1.,-1.E-15,-2.E-15));
#20388=DIRECTION('ref_axis',(-2.E-15,0.,-1.));
#20389=DIRECTION('',(2.E-15,-1.39036381887169E-17,1.));
#20390=DIRECTION('',(-2.E-15,2.94543590196345E-19,-1.));
#20391=DIRECTION('',(1.E-15,1.,2.94543590196345E-19));
#20392=DIRECTION('center_axis',(-2.E-15,2.94543590198344E-19,-1.));
#20393=DIRECTION('ref_axis',(1.E-15,1.,2.94543590196345E-19));
#20394=DIRECTION('',(1.,-1.E-15,-2.E-15));
#20395=DIRECTION('',(-1.,1.E-15,2.E-15));
#20396=DIRECTION('',(1.E-15,1.,2.94543590196345E-19));
#20397=DIRECTION('center_axis',(1.,-1.E-15,-2.E-15));
#20398=DIRECTION('ref_axis',(-2.E-15,0.,-1.));
#20399=DIRECTION('',(2.E-15,-1.39036381887169E-17,1.));
#20400=DIRECTION('',(-2.E-15,2.94543590196345E-19,-1.));
#20401=DIRECTION('',(1.E-15,1.,2.94543590196345E-19));
#20402=DIRECTION('center_axis',(-2.E-15,2.94543590198344E-19,-1.));
#20403=DIRECTION('ref_axis',(1.E-15,1.,2.94543590196345E-19));
#20404=DIRECTION('',(1.,-1.E-15,-2.E-15));
#20405=DIRECTION('',(-1.,1.E-15,2.E-15));
#20406=DIRECTION('',(1.E-15,1.,2.94543590196345E-19));
#20407=DIRECTION('center_axis',(1.,-1.E-15,-2.E-15));
#20408=DIRECTION('ref_axis',(-2.E-15,0.,-1.));
#20409=DIRECTION('',(2.E-15,-1.39036381887169E-17,1.));
#20410=DIRECTION('',(-2.E-15,2.94543590196345E-19,-1.));
#20411=DIRECTION('',(1.E-15,1.,2.94543590196345E-19));
#20412=DIRECTION('center_axis',(-2.E-15,2.94543590198344E-19,-1.));
#20413=DIRECTION('ref_axis',(1.E-15,1.,2.94543590196345E-19));
#20414=DIRECTION('',(1.,-1.E-15,-2.E-15));
#20415=DIRECTION('',(-1.,1.E-15,2.E-15));
#20416=DIRECTION('',(1.E-15,1.,2.94543590196345E-19));
#20417=DIRECTION('center_axis',(-2.E-15,2.94543590198344E-19,-1.));
#20418=DIRECTION('ref_axis',(1.E-15,1.,2.94543590196345E-19));
#20419=DIRECTION('',(1.,-1.E-15,-2.E-15));
#20420=DIRECTION('',(1.E-15,1.,2.94543590196345E-19));
#20421=DIRECTION('',(-1.,1.E-15,2.E-15));
#20422=DIRECTION('',(1.E-15,1.,2.94543590196345E-19));
#20423=DIRECTION('center_axis',(-1.,1.E-15,2.E-15));
#20424=DIRECTION('ref_axis',(-1.E-15,-1.,1.44148758291472E-46));
#20425=DIRECTION('',(-2.E-15,1.39036381887169E-17,-1.));
#20426=DIRECTION('',(1.E-15,1.,2.94543590196345E-19));
#20427=DIRECTION('',(2.E-15,-2.94543590196345E-19,1.));
#20428=DIRECTION('',(1.E-15,1.,2.94543590196345E-19));
#20429=DIRECTION('center_axis',(2.10217463002298E-15,-2.94543590198447E-19,
1.));
#20430=DIRECTION('ref_axis',(1.E-15,1.,2.94543590196345E-19));
#20431=DIRECTION('',(-1.,1.E-15,2.10217463002298E-15));
#20432=DIRECTION('',(1.,-1.E-15,-2.10217463002298E-15));
#20433=DIRECTION('',(1.E-15,1.,2.94543590196345E-19));
#20434=DIRECTION('center_axis',(-2.E-15,2.94543590198344E-19,-1.));
#20435=DIRECTION('ref_axis',(1.E-15,1.,2.94543590196345E-19));
#20436=DIRECTION('',(1.,-1.E-15,-2.E-15));
#20437=DIRECTION('',(1.E-15,1.,2.94543590196345E-19));
#20438=DIRECTION('',(-1.,1.E-15,2.E-15));
#20439=DIRECTION('center_axis',(-1.,1.E-15,1.25746720174781E-15));
#20440=DIRECTION('ref_axis',(-1.E-15,-1.,9.45020606069163E-47));
#20441=DIRECTION('',(-1.E-15,-1.,-1.88507897725893E-17));
#20442=DIRECTION('',(-1.E-15,-1.,-1.88507897725893E-17));
#20443=DIRECTION('center_axis',(1.,-1.E-15,-1.25746720174781E-15));
#20444=DIRECTION('ref_axis',(-1.25746720174781E-15,-7.42532798252193E-31,
-1.));
#20445=DIRECTION('',(-1.E-15,-1.,-1.88507897725893E-17));
#20446=DIRECTION('',(-1.E-15,-1.,-1.88507897725893E-17));
#20447=DIRECTION('center_axis',(2.E-15,-1.88507897725913E-17,1.));
#20448=DIRECTION('ref_axis',(1.E-15,1.,1.88507897725894E-17));
#20449=DIRECTION('',(-1.,1.E-15,2.E-15));
#20450=DIRECTION('',(-1.E-15,-1.,-1.88507897725893E-17));
#20451=DIRECTION('',(-1.,1.E-15,2.E-15));
#20452=DIRECTION('center_axis',(-2.E-15,1.88507897725913E-17,-1.));
#20453=DIRECTION('ref_axis',(1.E-15,1.,1.88507897725894E-17));
#20454=DIRECTION('',(-1.E-15,-1.,-1.88507897725893E-17));
#20455=DIRECTION('',(-1.E-15,-1.,-1.88507897725893E-17));
#20456=DIRECTION('',(1.,-1.E-15,-2.E-15));
#20457=DIRECTION('center_axis',(1.,-1.E-15,-2.E-15));
#20458=DIRECTION('ref_axis',(-2.E-15,0.,-1.));
#20459=DIRECTION('',(-1.E-15,-1.,-1.88507897725893E-17));
#20460=DIRECTION('center_axis',(2.E-15,-1.88507897725913E-17,1.));
#20461=DIRECTION('ref_axis',(1.E-15,1.,1.88507897725894E-17));
#20462=DIRECTION('',(-1.E-15,-1.,-1.88507897725893E-17));
#20463=DIRECTION('',(-1.,1.E-15,2.E-15));
#20464=DIRECTION('center_axis',(-1.,1.E-15,2.E-15));
#20465=DIRECTION('ref_axis',(-1.E-15,-1.,1.44148758291472E-46));
#20466=DIRECTION('',(2.E-15,-1.39036381887169E-17,1.));
#20467=DIRECTION('',(1.E-15,1.,1.0891631049783E-16));
#20468=DIRECTION('',(-2.E-15,4.20505361484229E-17,-1.));
#20469=DIRECTION('center_axis',(-1.,1.E-15,2.E-15));
#20470=DIRECTION('ref_axis',(2.E-15,-2.E-30,1.));
#20471=DIRECTION('center_axis',(-1.,1.E-15,2.E-15));
#20472=DIRECTION('ref_axis',(2.E-15,-2.E-30,1.));
#20473=DIRECTION('',(1.,-1.E-15,-2.E-15));
#20474=DIRECTION('center_axis',(1.,-1.E-15,-2.E-15));
#20475=DIRECTION('ref_axis',(2.E-15,-2.E-30,1.));
#20476=DIRECTION('',(-1.,1.E-15,2.E-15));
#20477=DIRECTION('center_axis',(-1.,1.E-15,2.E-15));
#20478=DIRECTION('ref_axis',(2.E-15,-2.E-30,1.));
#20479=DIRECTION('center_axis',(-1.,1.E-15,2.E-15));
#20480=DIRECTION('ref_axis',(2.E-15,-2.E-30,1.));
#20481=DIRECTION('',(1.,-1.E-15,-2.E-15));
#20482=DIRECTION('center_axis',(1.,-1.E-15,-2.E-15));
#20483=DIRECTION('ref_axis',(2.E-15,-2.E-30,1.));
#20484=DIRECTION('',(-1.,1.E-15,2.E-15));
#20485=DIRECTION('center_axis',(1.,-1.E-15,-2.E-15));
#20486=DIRECTION('ref_axis',(-2.E-15,2.E-30,-1.));
#20487=DIRECTION('center_axis',(-1.,1.E-15,2.E-15));
#20488=DIRECTION('ref_axis',(2.E-15,-2.E-30,1.));
#20489=DIRECTION('',(1.,-1.E-15,-2.E-15));
#20490=DIRECTION('center_axis',(1.,-1.E-15,-2.E-15));
#20491=DIRECTION('ref_axis',(2.E-15,-2.E-30,1.));
#20492=DIRECTION('',(-1.,1.E-15,2.E-15));
#20493=DIRECTION('center_axis',(1.,-1.E-15,-2.E-15));
#20494=DIRECTION('ref_axis',(-2.E-15,2.E-30,-1.));
#20495=DIRECTION('center_axis',(-1.,1.E-15,2.E-15));
#20496=DIRECTION('ref_axis',(2.E-15,-2.E-30,1.));
#20497=DIRECTION('',(1.,-1.E-15,-2.E-15));
#20498=DIRECTION('center_axis',(1.,-1.E-15,-2.E-15));
#20499=DIRECTION('ref_axis',(2.E-15,-2.E-30,1.));
#20500=DIRECTION('',(-1.,1.E-15,2.E-15));
#20501=DIRECTION('center_axis',(2.E-15,-1.39036381887169E-17,1.));
#20502=DIRECTION('ref_axis',(-2.78072763774338E-32,-1.,-1.39036381887169E-17));
#20503=DIRECTION('',(2.E-15,-1.39036381887169E-17,1.));
#20504=DIRECTION('',(-2.E-15,1.39036381887169E-17,-1.));
#20505=DIRECTION('',(2.E-15,-1.39036381887169E-17,1.));
#20506=DIRECTION('',(2.E-15,0.,1.));
#20507=DIRECTION('center_axis',(2.E-15,0.,1.));
#20508=DIRECTION('ref_axis',(1.,-1.E-15,-2.E-15));
#20509=DIRECTION('',(1.E-15,1.,0.));
#20510=DIRECTION('',(1.E-15,1.,0.));
#20511=DIRECTION('center_axis',(1.E-15,1.,-2.E-30));
#20512=DIRECTION('ref_axis',(-2.E-15,1.44148758291472E-46,-1.));
#20513=DIRECTION('center_axis',(-2.E-15,2.E-30,-1.));
#20514=DIRECTION('ref_axis',(1.E-15,1.,0.));
#20515=DIRECTION('',(-1.E-15,-1.,0.));
#20516=DIRECTION('',(-1.E-15,-1.,0.));
#20517=DIRECTION('center_axis',(-1.,1.E-15,2.E-15));
#20518=DIRECTION('ref_axis',(-1.E-15,-1.,1.44148758291472E-46));
#20519=DIRECTION('',(-2.E-15,2.94543590196345E-19,-1.));
#20520=DIRECTION('center_axis',(-1.,1.E-15,2.E-15));
#20521=DIRECTION('ref_axis',(-1.E-15,-1.,1.44148758291472E-46));
#20522=DIRECTION('center_axis',(-2.E-15,2.E-30,-1.));
#20523=DIRECTION('ref_axis',(1.E-15,1.,0.));
#20524=DIRECTION('',(-1.,1.E-15,2.E-15));
#20525=DIRECTION('',(1.E-15,1.,0.));
#20526=DIRECTION('center_axis',(2.E-15,0.,1.));
#20527=DIRECTION('ref_axis',(1.,-1.E-15,-2.E-15));
#20528=DIRECTION('',(-1.E-15,-1.,0.));
#20529=DIRECTION('',(1.,-1.E-15,-2.E-15));
#20530=DIRECTION('center_axis',(-1.E-15,-1.,0.));
#20531=DIRECTION('ref_axis',(-1.,1.E-15,2.E-15));
#20532=DIRECTION('',(-1.,1.E-15,2.E-15));
#20533=DIRECTION('',(2.E-15,0.,1.));
#20534=DIRECTION('',(1.,-1.E-15,-2.E-15));
#20535=DIRECTION('',(2.E-15,0.,1.));
#20536=DIRECTION('center_axis',(1.,-1.E-15,-2.E-15));
#20537=DIRECTION('ref_axis',(-2.E-15,0.,-1.));
#20538=DIRECTION('center_axis',(-1.,1.E-15,2.E-15));
#20539=DIRECTION('ref_axis',(-2.E-15,-1.93999646477936E-30,-1.));
#20540=DIRECTION('',(-2.E-15,2.11758236813575E-19,-1.));
#20541=DIRECTION('',(2.E-15,-1.39036381887169E-17,1.));
#20542=DIRECTION('center_axis',(1.,-1.E-15,-2.E-15));
#20543=DIRECTION('ref_axis',(-2.E-15,-1.22385608907605E-30,-1.));
#20544=DIRECTION('center_axis',(-1.,1.57824115865894E-15,2.E-15));
#20545=DIRECTION('ref_axis',(2.E-15,0.,1.));
#20546=DIRECTION('center_axis',(-1.,1.40298201113451E-15,2.E-15));
#20547=DIRECTION('ref_axis',(1.40298201113451E-15,1.,-2.80596402226901E-30));
#20548=DIRECTION('',(-2.E-15,1.39036381887169E-17,-1.));
#20549=DIRECTION('',(2.E-15,-2.11758236813575E-19,1.));
#20550=DIRECTION('center_axis',(1.,-1.49249955809742E-15,-2.E-15));
#20551=DIRECTION('ref_axis',(1.49249955809742E-15,1.,-2.98499911619484E-30));
#20552=DIRECTION('center_axis',(-8.78027255595381E-16,-1.,1.75605451119076E-30));
#20553=DIRECTION('ref_axis',(2.E-15,1.65592381969512E-47,1.));
#20554=DIRECTION('',(-1.,1.E-15,2.E-15));
#20555=DIRECTION('',(2.E-15,0.,1.));
#20556=DIRECTION('',(1.,-8.78027255595381E-16,-2.E-15));
#20557=DIRECTION('',(2.E-15,0.,1.));
#20558=DIRECTION('center_axis',(1.,-1.E-15,-2.E-15));
#20559=DIRECTION('ref_axis',(-2.E-15,0.,-1.));
#20560=DIRECTION('center_axis',(-1.,1.E-15,2.E-15));
#20561=DIRECTION('ref_axis',(-2.E-15,3.00017676103224E-32,-1.));
#20562=DIRECTION('',(-2.E-15,2.11758236813575E-19,-1.));
#20563=DIRECTION('',(2.E-15,-1.39036381887169E-17,1.));
#20564=DIRECTION('center_axis',(1.,-1.E-15,-2.E-15));
#20565=DIRECTION('ref_axis',(-2.E-15,3.88071955461975E-31,-1.));
#20566=DIRECTION('center_axis',(-1.,1.E-15,2.E-15));
#20567=DIRECTION('ref_axis',(-1.E-15,-1.,1.44148758291472E-46));
#20568=DIRECTION('',(-2.E-15,2.492418787323E-17,-1.));
#20569=DIRECTION('',(2.E-15,-2.11758236813575E-19,1.));
#20570=DIRECTION('center_axis',(1.,-1.E-15,-2.E-15));
#20571=DIRECTION('ref_axis',(2.E-15,-3.93999646477935E-15,1.));
#20572=DIRECTION('center_axis',(-1.,1.E-15,2.E-15));
#20573=DIRECTION('ref_axis',(2.E-15,1.22385608907605E-30,1.));
#20574=DIRECTION('center_axis',(2.E-15,0.,1.));
#20575=DIRECTION('ref_axis',(1.,0.,-2.E-15));
#20576=DIRECTION('',(2.E-15,0.,1.));
#20577=DIRECTION('center_axis',(2.E-15,0.,1.));
#20578=DIRECTION('ref_axis',(1.,0.,-2.E-15));
#20579=DIRECTION('',(2.E-15,0.,1.));
#20580=DIRECTION('center_axis',(2.E-15,-1.35525271560688E-16,1.));
#20581=DIRECTION('ref_axis',(2.71050543121376E-31,1.,1.35525271560688E-16));
#20582=DIRECTION('center_axis',(-1.,1.E-15,2.E-15));
#20583=DIRECTION('ref_axis',(-1.E-15,-1.,1.44148758291472E-46));
#20584=DIRECTION('',(2.E-15,0.,1.));
#20585=DIRECTION('',(-1.E-15,-1.,0.));
#20586=DIRECTION('',(-1.E-15,-1.,-1.0891631049783E-16));
#20587=DIRECTION('center_axis',(2.E-15,0.,1.));
#20588=DIRECTION('ref_axis',(1.,0.,-2.E-15));
#20589=DIRECTION('',(2.E-15,0.,1.));
#20590=DIRECTION('center_axis',(2.E-15,0.,1.));
#20591=DIRECTION('ref_axis',(1.,0.,-2.E-15));
#20592=DIRECTION('center_axis',(2.E-15,-1.35525271560688E-16,1.));
#20593=DIRECTION('ref_axis',(2.71050543121376E-31,1.,1.35525271560688E-16));
#20594=DIRECTION('center_axis',(1.,-1.E-15,-2.E-15));
#20595=DIRECTION('ref_axis',(-2.E-15,0.,-1.));
#20596=DIRECTION('',(1.E-15,1.,0.));
#20597=DIRECTION('',(1.E-15,1.,1.0891631049783E-16));
#20598=DIRECTION('center_axis',(2.E-15,0.,1.));
#20599=DIRECTION('ref_axis',(1.,0.,-2.E-15));
#20600=DIRECTION('',(2.E-15,0.,1.));
#20601=DIRECTION('center_axis',(2.E-15,0.,1.));
#20602=DIRECTION('ref_axis',(1.,0.,-2.E-15));
#20603=DIRECTION('',(2.E-15,0.,1.));
#20604=DIRECTION('center_axis',(2.E-15,-1.35525271560688E-16,1.));
#20605=DIRECTION('ref_axis',(1.0842021724855E-15,1.,1.35525271560686E-16));
#20606=DIRECTION('center_axis',(-1.,1.E-15,2.E-15));
#20607=DIRECTION('ref_axis',(-1.E-15,-1.,1.44148758291472E-46));
#20608=DIRECTION('',(2.E-15,0.,1.));
#20609=DIRECTION('',(-1.E-15,-1.,0.));
#20610=DIRECTION('',(-1.E-15,-1.,-1.0891631049783E-16));
#20611=DIRECTION('center_axis',(2.E-15,0.,1.));
#20612=DIRECTION('ref_axis',(1.,0.,-2.E-15));
#20613=DIRECTION('',(2.E-15,0.,1.));
#20614=DIRECTION('center_axis',(2.E-15,0.,1.));
#20615=DIRECTION('ref_axis',(1.,0.,-2.E-15));
#20616=DIRECTION('center_axis',(2.E-15,-1.35525271560688E-16,1.));
#20617=DIRECTION('ref_axis',(1.0842021724855E-15,1.,1.35525271560686E-16));
#20618=DIRECTION('center_axis',(1.,-1.E-15,-2.E-15));
#20619=DIRECTION('ref_axis',(-2.E-15,0.,-1.));
#20620=DIRECTION('',(1.E-15,1.,0.));
#20621=DIRECTION('',(1.E-15,1.,1.0891631049783E-16));
#20622=DIRECTION('center_axis',(-1.,1.E-15,2.E-15));
#20623=DIRECTION('ref_axis',(-1.E-15,-1.,1.44148758291472E-46));
#20624=DIRECTION('center_axis',(1.,-1.E-15,-2.E-15));
#20625=DIRECTION('ref_axis',(2.E-15,-3.93999646477936E-15,1.));
#20626=DIRECTION('',(-1.E-15,-1.,0.));
#20627=DIRECTION('',(2.E-15,0.,1.));
#20628=DIRECTION('',(-1.E-15,-1.,-1.0891631049783E-16));
#20629=DIRECTION('',(-1.E-15,-1.,-1.0891631049783E-16));
#20630=DIRECTION('center_axis',(-2.E-15,1.08916310497832E-16,-1.));
#20631=DIRECTION('ref_axis',(1.E-15,1.,1.0891631049783E-16));
#20632=DIRECTION('',(-1.,1.E-15,2.E-15));
#20633=DIRECTION('',(1.,-1.E-15,-2.E-15));
#20634=DIRECTION('',(1.E-15,1.,1.0891631049783E-16));
#20635=DIRECTION('center_axis',(1.,-1.E-15,-2.E-15));
#20636=DIRECTION('ref_axis',(-2.E-15,0.,-1.));
#20637=DIRECTION('',(-2.E-15,4.20505361484229E-17,-1.));
#20638=DIRECTION('center_axis',(-1.,1.E-15,2.E-15));
#20639=DIRECTION('ref_axis',(2.E-15,1.49100556725305E-32,1.));
#20640=DIRECTION('center_axis',(-2.E-15,1.08916310497832E-16,-1.));
#20641=DIRECTION('ref_axis',(1.E-15,1.,1.0891631049783E-16));
#20642=DIRECTION('',(1.,-1.E-15,-2.E-15));
#20643=DIRECTION('',(1.E-15,1.,1.0891631049783E-16));
#20644=DIRECTION('',(1.,-1.E-15,-2.E-15));
#20645=DIRECTION('center_axis',(1.,-1.E-15,-2.E-15));
#20646=DIRECTION('ref_axis',(-2.E-15,2.E-30,-1.));
#20647=DIRECTION('',(1.,-1.E-15,-2.E-15));
#20648=DIRECTION('',(1.,-1.E-15,-2.E-15));
#20649=DIRECTION('center_axis',(-1.,1.E-15,2.E-15));
#20650=DIRECTION('ref_axis',(2.E-15,-2.E-30,1.));
#20651=DIRECTION('center_axis',(-1.E-15,-1.,-1.39036381887169E-17));
#20652=DIRECTION('ref_axis',(-1.,1.E-15,2.E-15));
#20653=DIRECTION('',(-2.E-15,1.39036381887169E-17,-1.));
#20654=DIRECTION('',(1.,-1.E-15,-2.E-15));
#20655=DIRECTION('',(-2.E-15,1.39036381887169E-17,-1.));
#20656=DIRECTION('',(-2.E-15,1.39036381887169E-17,-1.));
#20657=DIRECTION('center_axis',(-2.E-15,2.E-30,-1.));
#20658=DIRECTION('ref_axis',(1.E-15,1.,0.));
#20659=DIRECTION('',(1.E-15,1.,0.));
#20660=DIRECTION('',(1.,-1.E-15,-2.E-15));
#20661=DIRECTION('center_axis',(1.E-15,1.,2.11758236811575E-19));
#20662=DIRECTION('ref_axis',(-2.E-15,2.11758236813575E-19,-1.));
#20663=DIRECTION('',(2.E-15,-2.11758236813575E-19,1.));
#20664=DIRECTION('',(1.,-1.E-15,-2.E-15));
#20665=DIRECTION('',(2.E-15,-2.11758236813575E-19,1.));
#20666=DIRECTION('',(2.E-15,-2.11758236813575E-19,1.));
#20667=DIRECTION('',(-2.E-15,2.94543590196345E-19,-1.));
#20668=DIRECTION('',(1.,-1.E-15,-2.E-15));
#20669=DIRECTION('',(1.,-1.E-15,-2.E-15));
#20670=DIRECTION('center_axis',(1.,-1.E-15,-2.E-15));
#20671=DIRECTION('ref_axis',(-2.E-15,2.E-30,-1.));
#20672=DIRECTION('',(1.,-1.E-15,-2.E-15));
#20673=DIRECTION('center_axis',(2.E-15,0.,1.));
#20674=DIRECTION('ref_axis',(1.,-1.E-15,-2.E-15));
#20675=DIRECTION('',(1.,-1.E-15,-2.E-15));
#20676=DIRECTION('',(1.,-1.E-15,-2.E-15));
#20677=DIRECTION('',(-1.E-15,-1.,0.));
#20678=DIRECTION('',(1.,-1.E-15,-2.E-15));
#20679=DIRECTION('center_axis',(-1.E-15,-1.,0.));
#20680=DIRECTION('ref_axis',(-1.,1.E-15,2.E-15));
#20681=DIRECTION('',(-2.E-15,0.,-1.));
#20682=DIRECTION('center_axis',(1.,-1.E-15,-2.E-15));
#20683=DIRECTION('ref_axis',(-2.E-15,2.E-30,-1.));
#20684=DIRECTION('center_axis',(1.,-1.E-15,-2.E-15));
#20685=DIRECTION('ref_axis',(-2.E-15,2.E-30,-1.));
#20686=DIRECTION('center_axis',(1.,-1.E-15,-2.E-15));
#20687=DIRECTION('ref_axis',(-2.E-15,2.E-30,-1.));
#20688=DIRECTION('center_axis',(1.,-1.E-15,-2.E-15));
#20689=DIRECTION('ref_axis',(-2.E-15,0.,-1.));
#20690=DIRECTION('center_axis',(1.,-1.E-15,-2.E-15));
#20691=DIRECTION('ref_axis',(-2.E-15,0.,-1.));
#20692=DIRECTION('center_axis',(1.,-1.E-15,-2.E-15));
#20693=DIRECTION('ref_axis',(-2.E-15,0.,-1.));
#20694=DIRECTION('center_axis',(-1.,1.E-15,2.E-15));
#20695=DIRECTION('ref_axis',(-1.E-15,-1.,1.44148758291472E-46));
#20696=DIRECTION('center_axis',(-1.,1.E-15,2.E-15));
#20697=DIRECTION('ref_axis',(-1.E-15,-1.,1.44148758291472E-46));
#20698=DIRECTION('center_axis',(-1.,1.E-15,2.E-15));
#20699=DIRECTION('ref_axis',(-1.E-15,-1.,1.44148758291472E-46));
#25002=CARTESIAN_POINT('',(0.,0.,0.));
#25003=CARTESIAN_POINT('Origin',(-31.761699248248,37.153679903937,214.471369141518));
#25004=CARTESIAN_POINT('',(-32.261699248248,37.153679903937,214.471369141518));
#25005=CARTESIAN_POINT('',(-31.761699248248,37.653679903937,213.971369141518));
#25006=CARTESIAN_POINT('Origin',(-31.76169924825,37.1536799039392,213.97136914152));
#25007=CARTESIAN_POINT('',(-31.261699248248,37.153679903937,214.471369141518));
#25008=CARTESIAN_POINT('Origin',(-31.7616992482473,37.1536799039377,213.971369141519));
#25009=CARTESIAN_POINT('',(-31.261699248248,37.153679903937,205.771369141518));
#25010=CARTESIAN_POINT('',(-31.261699248248,37.153679903937,214.471369141518));
#25011=CARTESIAN_POINT('',(-31.761699248248,37.653679903937,206.271369141518));
#25012=CARTESIAN_POINT('Origin',(-31.7616992482484,37.1536799039366,206.271369141519));
#25013=CARTESIAN_POINT('',(-32.261699248248,37.153679903937,205.771369141518));
#25014=CARTESIAN_POINT('Origin',(-31.761699248248,37.1536799039369,206.271369141518));
#25015=CARTESIAN_POINT('',(-32.261699248248,37.153679903937,214.471369141518));
#25016=CARTESIAN_POINT('Origin',(-32.261699248248,37.153679903937,206.271369141518));
#25017=CARTESIAN_POINT('',(-32.261699248248,37.153679903937,205.771369141518));
#25018=CARTESIAN_POINT('Origin',(-32.261699248248,37.153679903937,213.971369141518));
#25019=CARTESIAN_POINT('',(-32.261699248248,37.153679903937,214.471369141518));
#25020=CARTESIAN_POINT('Origin',(1.93830075175198,37.1536799039369,207.844898865397));
#25021=CARTESIAN_POINT('',(1.43830075175198,37.1536799039369,207.844898865397));
#25022=CARTESIAN_POINT('',(1.93830075175198,37.6536799039369,207.344898865397));
#25023=CARTESIAN_POINT('Origin',(1.93830075175113,37.1536799039378,207.344898865398));
#25024=CARTESIAN_POINT('',(2.43830075175198,37.1536799039369,207.844898865397));
#25025=CARTESIAN_POINT('Origin',(1.93830075175171,37.1536799039367,207.344898865397));
#25026=CARTESIAN_POINT('',(2.43830075175197,37.1536799039369,198.5));
#25027=CARTESIAN_POINT('',(2.43830075175198,37.1536799039369,207.844898865397));
#25028=CARTESIAN_POINT('',(1.93830075175197,37.6536799039369,199.));
#25029=CARTESIAN_POINT('Origin',(1.93830075175225,37.1536799039372,199.));
#25030=CARTESIAN_POINT('',(1.43830075175197,37.1536799039369,198.5));
#25031=CARTESIAN_POINT('Origin',(1.93830075175189,37.153679903937,199.));
#25032=CARTESIAN_POINT('',(1.43830075175198,37.1536799039369,207.844898865397));
#25033=CARTESIAN_POINT('Origin',(-69.261699248248,37.153679903937,199.));
#25034=CARTESIAN_POINT('',(-69.261699248248,37.153679903937,198.5));
#25035=CARTESIAN_POINT('Origin',(1.43830075175198,37.1536799039369,207.344898865397));
#25036=CARTESIAN_POINT('',(1.43830075175198,37.1536799039369,207.844898865397));
#25037=CARTESIAN_POINT('Origin',(1.938300751752,37.1536799039369,214.501561642103));
#25038=CARTESIAN_POINT('',(1.438300751752,37.1536799039369,214.501561642103));
#25039=CARTESIAN_POINT('',(1.938300751752,37.6536799039369,214.001561642103));
#25040=CARTESIAN_POINT('Origin',(1.93830075175188,37.1536799039369,214.001561642103));
#25041=CARTESIAN_POINT('',(2.438300751752,37.1536799039369,214.501561642103));
#25042=CARTESIAN_POINT('Origin',(1.93830075175259,37.1536799039376,214.001561642104));
#25043=CARTESIAN_POINT('',(2.43830075175199,37.1536799039369,209.344898865397));
#25044=CARTESIAN_POINT('',(2.438300751752,37.1536799039369,214.501561642103));
#25045=CARTESIAN_POINT('',(1.93830075175199,37.6536799039369,209.844898865397));
#25046=CARTESIAN_POINT('Origin',(1.93830075175128,37.1536799039362,209.844898865398));
#25047=CARTESIAN_POINT('',(1.43830075175199,37.1536799039369,209.344898865397));
#25048=CARTESIAN_POINT('Origin',(1.93830075175241,37.1536799039365,209.844898865398));
#25049=CARTESIAN_POINT('',(1.438300751752,37.1536799039369,214.501561642103));
#25050=CARTESIAN_POINT('Origin',(1.43830075175199,37.1536799039369,209.844898865397));
#25051=CARTESIAN_POINT('',(1.43830075175199,37.1536799039369,209.344898865397));
#25052=CARTESIAN_POINT('Origin',(1.438300751752,37.1536799039369,214.001561642103));
#25053=CARTESIAN_POINT('',(1.438300751752,37.1536799039369,214.501561642103));
#25054=CARTESIAN_POINT('Ctrl Pts',(-69.761699248248,33.353679903937,209.3));
#25055=CARTESIAN_POINT('Ctrl Pts',(-69.761699248248,32.853679903937,209.3));
#25056=CARTESIAN_POINT('Ctrl Pts',(-69.261699248248,32.853679903937,209.3));
#25057=CARTESIAN_POINT('Ctrl Pts',(-70.261699248248,33.353679903937,209.3));
#25058=CARTESIAN_POINT('Ctrl Pts',(-70.261699248248,32.353679903937,209.3));
#25059=CARTESIAN_POINT('Ctrl Pts',(-69.261699248248,32.353679903937,209.3));
#25060=CARTESIAN_POINT('Ctrl Pts',(-70.261699248248,33.353679903937,209.8));
#25061=CARTESIAN_POINT('Ctrl Pts',(-70.261699248248,32.353679903937,209.8));
#25062=CARTESIAN_POINT('Ctrl Pts',(-69.261699248248,32.353679903937,209.8));
#25063=CARTESIAN_POINT('',(-69.261699248248,32.353679903937,209.8));
#25064=CARTESIAN_POINT('',(-69.261699248248,32.853679903937,209.3));
#25065=CARTESIAN_POINT('Origin',(-69.261699248248,32.853679903937,209.8));
#25066=CARTESIAN_POINT('',(-70.261699248248,33.353679903937,209.8));
#25067=CARTESIAN_POINT('Origin',(-69.261699248248,33.353679903937,209.8));
#25068=CARTESIAN_POINT('',(-69.761699248248,33.353679903937,209.3));
#25069=CARTESIAN_POINT('Origin',(-69.761699248248,33.353679903937,209.8));
#25070=CARTESIAN_POINT('Origin',(-69.261699248248,33.353679903937,209.3));
#25071=CARTESIAN_POINT('Origin',(-69.761699248248,33.353679903937,209.8));
#25072=CARTESIAN_POINT('',(-70.261699248248,35.053679903937,209.8));
#25073=CARTESIAN_POINT('',(-69.261699248248,35.053679903937,209.8));
#25074=CARTESIAN_POINT('Origin',(-69.761699248248,35.053679903937,209.8));
#25075=CARTESIAN_POINT('',(-69.261699248248,33.353679903937,209.8));
#25076=CARTESIAN_POINT('',(-69.261699248248,35.553679903937,209.8));
#25077=CARTESIAN_POINT('Origin',(-69.761699248248,33.353679903937,209.8));
#25078=CARTESIAN_POINT('',(-70.261699248248,33.353679903937,209.8));
#25079=CARTESIAN_POINT('Origin',(-69.761699248248,35.053679903937,209.8));
#25080=CARTESIAN_POINT('Origin',(-69.761699248248,35.053679903937,209.8));
#25081=CARTESIAN_POINT('Origin',(-69.761699248248,35.053679903937,215.5));
#25082=CARTESIAN_POINT('',(-70.261699248248,35.053679903937,214.));
#25083=CARTESIAN_POINT('',(-69.261699248248,35.053679903937,214.));
#25084=CARTESIAN_POINT('Origin',(-69.761699248248,35.053679903937,214.));
#25085=CARTESIAN_POINT('',(-69.261699248248,35.053679903937,213.325088768032));
#25086=CARTESIAN_POINT('',(-69.261699248248,35.053679903937,209.3));
#25087=CARTESIAN_POINT('',(-69.261699248248,35.053679903937,210.465382311583));
#25088=CARTESIAN_POINT('',(-69.261699248248,35.053679903937,209.3));
#25089=CARTESIAN_POINT('',(-69.261699248248,35.053679903937,209.3));
#25090=CARTESIAN_POINT('',(-70.261699248248,35.053679903937,210.465382311583));
#25091=CARTESIAN_POINT('',(-70.261699248248,35.053679903937,209.8));
#25092=CARTESIAN_POINT('',(-70.261699248248,35.053679903937,213.325088768032));
#25093=CARTESIAN_POINT('',(-70.261699248248,35.053679903937,209.965382311583));
#25094=CARTESIAN_POINT('',(-70.261699248248,35.053679903937,209.8));
#25095=CARTESIAN_POINT('Origin',(-69.761699248248,35.053679903937,214.));
#25096=CARTESIAN_POINT('Origin',(-69.761699248248,35.053679903937,214.));
#25097=CARTESIAN_POINT('Origin',(-69.761699248248,33.353679903937,214.));
#25098=CARTESIAN_POINT('',(-70.261699248248,33.353679903937,214.));
#25099=CARTESIAN_POINT('',(-69.761699248248,33.353679903937,214.5));
#25100=CARTESIAN_POINT('Origin',(-69.761699248248,33.353679903937,214.));
#25101=CARTESIAN_POINT('',(-69.261699248248,33.353679903937,214.));
#25102=CARTESIAN_POINT('Origin',(-69.761699248248,33.353679903937,214.));
#25103=CARTESIAN_POINT('',(-69.261699248248,35.553679903937,214.));
#25104=CARTESIAN_POINT('',(-70.261699248248,35.053679903937,214.));
#25105=CARTESIAN_POINT('Ctrl Pts',(-69.261699248248,32.853679903937,214.5));
#25106=CARTESIAN_POINT('Ctrl Pts',(-69.761699248248,32.853679903937,214.5));
#25107=CARTESIAN_POINT('Ctrl Pts',(-69.761699248248,33.353679903937,214.5));
#25108=CARTESIAN_POINT('Ctrl Pts',(-69.261699248248,32.353679903937,214.5));
#25109=CARTESIAN_POINT('Ctrl Pts',(-70.261699248248,32.353679903937,214.5));
#25110=CARTESIAN_POINT('Ctrl Pts',(-70.261699248248,33.353679903937,214.5));
#25111=CARTESIAN_POINT('Ctrl Pts',(-69.261699248248,32.353679903937,214.));
#25112=CARTESIAN_POINT('Ctrl Pts',(-70.261699248248,32.353679903937,214.));
#25113=CARTESIAN_POINT('Ctrl Pts',(-70.261699248248,33.353679903937,214.));
#25114=CARTESIAN_POINT('',(-69.261699248248,32.353679903937,214.));
#25115=CARTESIAN_POINT('',(-69.261699248248,32.3608987452201,214.084656539108));
#25116=CARTESIAN_POINT('Origin',(-69.261699248248,32.853679903937,214.));
#25117=CARTESIAN_POINT('',(-69.261699248248,32.853679903937,214.5));
#25118=CARTESIAN_POINT('Origin',(-69.261699248248,32.853679903937,214.));
#25119=CARTESIAN_POINT('Origin',(-69.261699248248,33.353679903937,214.5));
#25120=CARTESIAN_POINT('Origin',(-69.261699248248,33.353679903937,214.));
#25121=CARTESIAN_POINT('Origin',(-70.261699248248,32.853679903937,214.));
#25122=CARTESIAN_POINT('',(-64.261699248248,32.3608987452201,214.084656539108));
#25123=CARTESIAN_POINT('',(-69.261699248248,32.3608987452201,214.084656539108));
#25124=CARTESIAN_POINT('',(-64.261699248248,32.353679903937,214.));
#25125=CARTESIAN_POINT('',(-70.261699248248,32.353679903937,214.));
#25126=CARTESIAN_POINT('Origin',(-64.261699248248,32.853679903937,214.));
#25127=CARTESIAN_POINT('Origin',(-32.561699248248,33.5567577319955,206.621369141518));
#25128=CARTESIAN_POINT('',(-32.261699248248,34.7567577319955,206.621369141518));
#25129=CARTESIAN_POINT('',(-32.261699248248,33.853679903937,206.621369141518));
#25130=CARTESIAN_POINT('',(-32.261699248248,37.653679903937,206.621369141518));
#25131=CARTESIAN_POINT('',(-32.3594092734667,33.5567577319955,206.621369141518));
#25132=CARTESIAN_POINT('Origin',(-32.761699248248,33.853679903937,206.621369141518));
#25133=CARTESIAN_POINT('',(-31.261699248248,33.5567577319955,206.621369141518));
#25134=CARTESIAN_POINT('',(-32.561699248248,33.5567577319955,206.621369141518));
#25135=CARTESIAN_POINT('',(-31.261699248248,34.7567577319955,206.621369141518));
#25136=CARTESIAN_POINT('',(-31.261699248248,33.5567577319955,206.621369141518));
#25137=CARTESIAN_POINT('',(-32.561699248248,34.7567577319955,206.621369141518));
#25138=CARTESIAN_POINT('Origin',(-32.561699248248,34.7567577319955,212.521369141518));
#25139=CARTESIAN_POINT('',(-32.261699248248,34.7567577319955,212.521369141518));
#25140=CARTESIAN_POINT('',(-32.261699248248,34.7567577319955,214.471369141518));
#25141=CARTESIAN_POINT('',(-31.261699248248,34.7567577319955,212.521369141518));
#25142=CARTESIAN_POINT('',(-31.261699248248,34.7567577319955,212.521369141518));
#25143=CARTESIAN_POINT('',(-32.561699248248,34.7567577319955,212.521369141518));
#25144=CARTESIAN_POINT('Origin',(-32.561699248248,36.2479932555265,212.521369141518));
#25145=CARTESIAN_POINT('',(-32.261699248248,36.2479932555265,212.521369141518));
#25146=CARTESIAN_POINT('',(-32.261699248248,37.653679903937,212.521369141518));
#25147=CARTESIAN_POINT('',(-31.261699248248,36.2479932555265,212.521369141518));
#25148=CARTESIAN_POINT('',(-31.261699248248,36.2479932555265,212.521369141518));
#25149=CARTESIAN_POINT('',(-32.561699248248,36.2479932555265,212.521369141518));
#25150=CARTESIAN_POINT('Origin',(-32.561699248248,36.2479932555265,213.621369141518));
#25151=CARTESIAN_POINT('',(-32.261699248248,36.2479932555265,213.621369141518));
#25152=CARTESIAN_POINT('',(-32.261699248248,36.2479932555265,214.471369141518));
#25153=CARTESIAN_POINT('',(-31.261699248248,36.2479932555265,213.621369141518));
#25154=CARTESIAN_POINT('',(-31.261699248248,36.2479932555265,213.621369141518));
#25155=CARTESIAN_POINT('',(-32.561699248248,36.2479932555265,213.621369141518));
#25156=CARTESIAN_POINT('Origin',(-32.561699248248,34.7567577319955,213.621369141518));
#25157=CARTESIAN_POINT('',(-32.261699248248,33.853679903937,213.621369141518));
#25158=CARTESIAN_POINT('',(-32.261699248248,37.653679903937,213.621369141518));
#25159=CARTESIAN_POINT('',(-31.261699248248,33.5567577319955,213.621369141518));
#25160=CARTESIAN_POINT('',(-31.261699248248,34.7567577319955,213.621369141518));
#25161=CARTESIAN_POINT('',(-32.3594092734667,33.5567577319955,213.621369141518));
#25162=CARTESIAN_POINT('',(-32.561699248248,33.5567577319955,213.621369141518));
#25163=CARTESIAN_POINT('Origin',(-32.761699248248,33.853679903937,213.621369141518));
#25164=CARTESIAN_POINT('Origin',(-32.561699248248,33.5567577319955,213.621369141518));
#25165=CARTESIAN_POINT('',(-31.261699248248,33.5567577319955,213.621369141518));
#25166=CARTESIAN_POINT('',(-32.3594092734667,33.5567577319955,214.471369141518));
#25167=CARTESIAN_POINT('Origin',(-31.761699248248,32.853679903937,198.5));
#25168=CARTESIAN_POINT('',(-31.261699248248,32.853679903937,205.771369141518));
#25169=CARTESIAN_POINT('',(-31.761699248248,32.353679903937,205.771369141518));
#25170=CARTESIAN_POINT('Origin',(-31.761699248248,32.853679903937,205.771369141518));
#25171=CARTESIAN_POINT('',(-31.261699248248,32.853679903937,214.471369141518));
#25172=CARTESIAN_POINT('',(-31.261699248248,32.853679903937,214.471369141518));
#25173=CARTESIAN_POINT('',(-31.761699248248,32.353679903937,214.471369141518));
#25174=CARTESIAN_POINT('Origin',(-31.761699248248,32.853679903937,214.471369141518));
#25175=CARTESIAN_POINT('',(-31.761699248248,32.353679903937,198.5));
#25176=CARTESIAN_POINT('Origin',(-32.761699248248,33.853679903937,214.471369141518));
#25177=CARTESIAN_POINT('',(-32.261699248248,33.853679903937,214.471369141518));
#25178=CARTESIAN_POINT('',(-32.261699248248,33.853679903937,214.471369141518));
#25179=CARTESIAN_POINT('',(-32.261699248248,33.853679903937,205.771369141518));
#25180=CARTESIAN_POINT('',(-32.261699248248,33.853679903937,214.471369141518));
#25181=CARTESIAN_POINT('',(-32.761699248248,33.353679903937,205.771369141518));
#25182=CARTESIAN_POINT('Origin',(-32.761699248248,33.853679903937,205.771369141518));
#25183=CARTESIAN_POINT('',(-32.761699248248,33.353679903937,214.471369141518));
#25184=CARTESIAN_POINT('',(-32.761699248248,33.353679903937,205.771369141518));
#25185=CARTESIAN_POINT('Origin',(-32.761699248248,33.853679903937,214.471369141518));
#25186=CARTESIAN_POINT('Origin',(-32.261699248248,37.653679903937,205.771369141518));
#25187=CARTESIAN_POINT('',(-32.261699248248,37.653679903937,205.771369141518));
#25188=CARTESIAN_POINT('',(-31.261699248248,37.653679903937,205.771369141518));
#25189=CARTESIAN_POINT('',(-32.261699248248,32.353679903937,205.771369141518));
#25190=CARTESIAN_POINT('',(-32.261699248248,32.353679903937,205.771369141518));
#25191=CARTESIAN_POINT('',(-32.261699248248,33.353679903937,205.771369141518));
#25192=CARTESIAN_POINT('',(-32.261699248248,32.2748332073222,205.771369141518));
#25193=CARTESIAN_POINT('',(-32.261699248248,33.353679903937,205.771369141518));
#25194=CARTESIAN_POINT('Origin',(-31.261699248248,37.653679903937,214.471369141518));
#25195=CARTESIAN_POINT('',(-31.261699248248,37.653679903937,214.471369141518));
#25196=CARTESIAN_POINT('Origin',(-32.261699248248,37.653679903937,214.471369141518));
#25197=CARTESIAN_POINT('',(-32.261699248248,37.653679903937,214.471369141518));
#25198=CARTESIAN_POINT('',(-32.261699248248,33.353679903937,214.471369141518));
#25199=CARTESIAN_POINT('',(-32.261699248248,33.353679903937,214.471369141518));
#25200=CARTESIAN_POINT('',(-32.261699248248,32.353679903937,214.471369141518));
#25201=CARTESIAN_POINT('',(-32.261699248248,32.2748332073222,214.471369141518));
#25202=CARTESIAN_POINT('',(-32.261699248248,32.353679903937,214.471369141518));
#25203=CARTESIAN_POINT('Origin',(-32.261699248248,37.653679903937,214.471369141518));
#25204=CARTESIAN_POINT('Origin',(1.93830075175196,32.8536799039369,198.5));
#25205=CARTESIAN_POINT('',(2.43830075175198,32.8536799039369,209.344898865397));
#25206=CARTESIAN_POINT('',(1.93830075175198,32.3536799039369,209.344898865397));
#25207=CARTESIAN_POINT('Origin',(1.93830075175198,32.8536799039369,209.344898865397));
#25208=CARTESIAN_POINT('',(2.438300751752,32.8536799039369,214.501561642103));
#25209=CARTESIAN_POINT('',(2.438300751752,32.8536799039369,214.501561642103));
#25210=CARTESIAN_POINT('',(1.938300751752,32.3536799039369,214.501561642103));
#25211=CARTESIAN_POINT('Origin',(1.938300751752,32.8536799039369,214.501561642103));
#25212=CARTESIAN_POINT('',(1.93830075175196,32.3536799039369,198.5));
#25213=CARTESIAN_POINT('Origin',(1.93830075175196,32.8536799039369,198.5));
#25214=CARTESIAN_POINT('',(2.43830075175196,32.8536799039369,198.5));
#25215=CARTESIAN_POINT('',(1.93830075175196,32.3536799039369,198.5));
#25216=CARTESIAN_POINT('Origin',(1.93830075175196,32.8536799039369,198.5));
#25217=CARTESIAN_POINT('',(2.43830075175198,32.8536799039369,207.844898865397));
#25218=CARTESIAN_POINT('',(2.43830075175198,32.8536799039369,207.844898865397));
#25219=CARTESIAN_POINT('',(1.93830075175198,32.3536799039369,207.844898865397));
#25220=CARTESIAN_POINT('Origin',(1.93830075175198,32.8536799039369,207.844898865397));
#25221=CARTESIAN_POINT('',(1.93830075175196,32.3536799039369,198.5));
#25222=CARTESIAN_POINT('Origin',(0.938300751751997,33.8536799039369,214.501561642103));
#25223=CARTESIAN_POINT('',(0.938300751751983,33.3536799039369,209.34762215292));
#25224=CARTESIAN_POINT('',(1.43830075175198,33.8536799039369,209.34762215292));
#25225=CARTESIAN_POINT('Origin',(0.938300751751983,33.8536799039369,209.34762215292));
#25226=CARTESIAN_POINT('',(0.938300751751997,33.3536799039369,214.5));
#25227=CARTESIAN_POINT('',(0.938300751751983,33.3536799039369,209.34762215292));
#25228=CARTESIAN_POINT('',(1.438300751752,33.8536799039369,214.5));
#25229=CARTESIAN_POINT('Origin',(0.938300751751997,33.8536799039369,214.5));
#25230=CARTESIAN_POINT('',(1.438300751752,33.8536799039369,214.5));
#25231=CARTESIAN_POINT('Origin',(0.938300751751983,33.8536799039369,207.844898865397));
#25232=CARTESIAN_POINT('',(0.938300751751962,33.3536799039369,198.5));
#25233=CARTESIAN_POINT('',(1.43830075175196,33.8536799039369,198.5));
#25234=CARTESIAN_POINT('Origin',(0.938300751751962,33.8536799039369,198.5));
#25235=CARTESIAN_POINT('',(0.938300751751983,33.3536799039369,207.844898865397));
#25236=CARTESIAN_POINT('',(0.938300751751962,33.3536799039369,198.5));
#25237=CARTESIAN_POINT('',(1.43830075175198,33.8536799039369,207.844898865397));
#25238=CARTESIAN_POINT('Origin',(0.938300751751983,33.8536799039369,207.844898865397));
#25239=CARTESIAN_POINT('',(1.43830075175198,33.8536799039369,207.844898865397));
#25240=CARTESIAN_POINT('Origin',(-16.261699248248,31.653679903937,209.34762215292));
#25241=CARTESIAN_POINT('',(-13.261699248248,32.3536799039369,209.34762215292));
#25242=CARTESIAN_POINT('',(-16.261699248248,32.353679903937,209.34762215292));
#25243=CARTESIAN_POINT('',(-69.261699248248,32.353679903937,209.34762215292));
#25244=CARTESIAN_POINT('',(-16.261699248248,33.353679903937,209.34762215292));
#25245=CARTESIAN_POINT('',(-16.261699248248,31.653679903937,209.34762215292));
#25246=CARTESIAN_POINT('',(-13.261699248248,33.3536799039369,209.34762215292));
#25247=CARTESIAN_POINT('',(-16.261699248248,33.353679903937,209.34762215292));
#25248=CARTESIAN_POINT('',(-13.261699248248,31.653679903937,209.34762215292));
#25249=CARTESIAN_POINT('Origin',(-13.261699248248,31.653679903937,209.34762215292));
#25250=CARTESIAN_POINT('',(-13.261699248248,32.3536799039369,207.84762215292));
#25251=CARTESIAN_POINT('',(-13.261699248248,32.3536799039369,198.5));
#25252=CARTESIAN_POINT('',(-13.261699248248,33.3536799039369,207.84762215292));
#25253=CARTESIAN_POINT('',(-13.261699248248,33.3536799039369,209.34762215292));
#25254=CARTESIAN_POINT('',(-13.261699248248,31.653679903937,207.84762215292));
#25255=CARTESIAN_POINT('Origin',(-13.261699248248,31.653679903937,207.84762215292));
#25256=CARTESIAN_POINT('',(-16.261699248248,32.353679903937,207.84762215292));
#25257=CARTESIAN_POINT('',(-69.261699248248,32.353679903937,207.84762215292));
#25258=CARTESIAN_POINT('',(-16.261699248248,33.353679903937,207.84762215292));
#25259=CARTESIAN_POINT('',(-13.261699248248,33.3536799039369,207.84762215292));
#25260=CARTESIAN_POINT('',(-16.261699248248,31.653679903937,207.84762215292));
#25261=CARTESIAN_POINT('Origin',(-16.261699248248,31.653679903937,207.84762215292));
#25262=CARTESIAN_POINT('',(-16.261699248248,32.353679903937,203.9));
#25263=CARTESIAN_POINT('',(-16.261699248248,32.353679903937,198.5));
#25264=CARTESIAN_POINT('',(-16.261699248248,33.353679903937,203.9));
#25265=CARTESIAN_POINT('',(-16.261699248248,33.353679903937,207.84762215292));
#25266=CARTESIAN_POINT('',(-16.261699248248,31.653679903937,203.9));
#25267=CARTESIAN_POINT('Origin',(-16.261699248248,31.653679903937,203.9));
#25268=CARTESIAN_POINT('',(-25.061699248248,32.353679903937,203.9));
#25269=CARTESIAN_POINT('',(-69.261699248248,32.353679903937,203.9));
#25270=CARTESIAN_POINT('',(-25.061699248248,33.353679903937,203.9));
#25271=CARTESIAN_POINT('',(-16.261699248248,33.353679903937,203.9));
#25272=CARTESIAN_POINT('',(-25.061699248248,31.653679903937,203.9));
#25273=CARTESIAN_POINT('Origin',(-25.061699248248,31.653679903937,203.9));
#25274=CARTESIAN_POINT('',(-25.061699248248,32.353679903937,201.4));
#25275=CARTESIAN_POINT('',(-25.061699248248,32.353679903937,198.5));
#25276=CARTESIAN_POINT('',(-25.061699248248,33.353679903937,201.4));
#25277=CARTESIAN_POINT('',(-25.061699248248,33.353679903937,203.9));
#25278=CARTESIAN_POINT('',(-25.061699248248,31.653679903937,201.4));
#25279=CARTESIAN_POINT('Origin',(-25.061699248248,31.653679903937,201.4));
#25280=CARTESIAN_POINT('',(-32.261699248248,32.353679903937,201.4));
#25281=CARTESIAN_POINT('',(-69.261699248248,32.353679903937,201.4));
#25282=CARTESIAN_POINT('',(-32.261699248248,33.353679903937,201.4));
#25283=CARTESIAN_POINT('',(-25.061699248248,33.353679903937,201.4));
#25284=CARTESIAN_POINT('',(-32.261699248248,31.653679903937,201.4));
#25285=CARTESIAN_POINT('Origin',(-35.261699248248,31.653679903937,210.957342646887));
#25286=CARTESIAN_POINT('',(-64.261699248248,32.353679903937,210.957342646887));
#25287=CARTESIAN_POINT('',(-35.261699248248,32.353679903937,210.957342646887));
#25288=CARTESIAN_POINT('',(-69.261699248248,32.353679903937,210.957342646887));
#25289=CARTESIAN_POINT('',(-35.261699248248,33.353679903937,210.957342646887));
#25290=CARTESIAN_POINT('',(-35.261699248248,31.653679903937,210.957342646887));
#25291=CARTESIAN_POINT('',(-64.261699248248,33.353679903937,210.957342646887));
#25292=CARTESIAN_POINT('',(-35.261699248248,33.353679903937,210.957342646887));
#25293=CARTESIAN_POINT('',(-64.261699248248,31.653679903937,210.957342646887));
#25294=CARTESIAN_POINT('Origin',(-7.05071200800411,31.6536799039369,207.84762215292));
#25295=CARTESIAN_POINT('',(-7.05071200800411,32.3536799039369,209.34762215292));
#25296=CARTESIAN_POINT('',(-7.05071200800411,32.3536799039369,207.84762215292));
#25297=CARTESIAN_POINT('',(-7.05071200800413,32.3536799039369,198.5));
#25298=CARTESIAN_POINT('',(-7.05071200800411,33.3536799039369,207.84762215292));
#25299=CARTESIAN_POINT('',(-7.05071200800411,31.6536799039369,207.84762215292));
#25300=CARTESIAN_POINT('',(-7.05071200800411,33.3536799039369,209.34762215292));
#25301=CARTESIAN_POINT('',(-7.05071200800411,33.3536799039369,207.84762215292));
#25302=CARTESIAN_POINT('',(-7.05071200800411,31.6536799039369,209.34762215292));
#25303=CARTESIAN_POINT('Origin',(1.43830075175198,31.6536799039369,209.34762215292));
#25304=CARTESIAN_POINT('',(1.43830075175198,32.3536799039369,209.34762215292));
#25305=CARTESIAN_POINT('',(-69.261699248248,32.353679903937,209.34762215292));
#25306=CARTESIAN_POINT('',(1.43830075175198,33.3536799039369,209.34762215292));
#25307=CARTESIAN_POINT('',(1.43830075175198,31.6536799039369,209.34762215292));
#25308=CARTESIAN_POINT('Origin',(1.43830075175198,31.6536799039369,207.84762215292));
#25309=CARTESIAN_POINT('',(1.43830075175198,32.3536799039369,207.84762215292));
#25310=CARTESIAN_POINT('',(-69.261699248248,32.353679903937,207.84762215292));
#25311=CARTESIAN_POINT('',(1.43830075175198,33.3536799039369,207.84762215292));
#25312=CARTESIAN_POINT('',(1.43830075175198,31.6536799039369,207.84762215292));
#25313=CARTESIAN_POINT('',(1.43830075175198,33.3536799039369,207.84762215292));
#25314=CARTESIAN_POINT('Origin',(1.43830075175198,37.6536799039369,207.844898865397));
#25315=CARTESIAN_POINT('',(1.43830075175198,37.6536799039369,207.844898865397));
#25316=CARTESIAN_POINT('',(1.43830075175197,37.6536799039369,198.5));
#25317=CARTESIAN_POINT('Origin',(2.43830075175198,37.6536799039369,207.844898865397));
#25318=CARTESIAN_POINT('',(2.43830075175197,37.6536799039369,198.5));
#25319=CARTESIAN_POINT('',(2.43830075175198,37.6536799039369,207.844898865397));
#25320=CARTESIAN_POINT('Origin',(1.43830075175198,37.6536799039369,207.844898865397));
#25321=CARTESIAN_POINT('',(1.43830075175198,33.3536799039369,207.844898865397));
#25322=CARTESIAN_POINT('',(1.43830075175198,33.3536799039369,207.844898865397));
#25323=CARTESIAN_POINT('',(1.43830075175198,32.3536799039369,207.844898865397));
#25324=CARTESIAN_POINT('',(1.43830075175198,37.6536799039369,207.844898865397));
#25325=CARTESIAN_POINT('',(1.43830075175198,32.3536799039369,207.844898865397));
#25326=CARTESIAN_POINT('Origin',(1.43830075175199,37.6536799039369,209.344898865397));
#25327=CARTESIAN_POINT('',(1.43830075175198,32.3536799039369,209.344898865397));
#25328=CARTESIAN_POINT('',(1.43830075175199,37.6536799039369,209.344898865397));
#25329=CARTESIAN_POINT('',(2.43830075175199,37.6536799039369,209.344898865397));
#25330=CARTESIAN_POINT('',(1.43830075175198,32.3536799039369,209.344898865397));
#25331=CARTESIAN_POINT('Origin',(2.438300751752,37.6536799039369,214.501561642103));
#25332=CARTESIAN_POINT('',(2.438300751752,37.6536799039369,214.501561642103));
#25333=CARTESIAN_POINT('Origin',(1.438300751752,37.6536799039369,214.501561642103));
#25334=CARTESIAN_POINT('',(1.438300751752,32.3536799039369,214.501561642103));
#25335=CARTESIAN_POINT('',(1.438300751752,37.6536799039369,214.501561642103));
#25336=CARTESIAN_POINT('',(1.438300751752,32.3536799039369,214.501561642103));
#25337=CARTESIAN_POINT('Origin',(1.438300751752,37.6536799039369,214.501561642103));
#25338=CARTESIAN_POINT('',(1.43830075175196,32.3536799039369,198.5));
#25339=CARTESIAN_POINT('',(1.438300751752,32.3536799039369,214.5));
#25340=CARTESIAN_POINT('',(1.43830075175199,31.72644166258,214.5));
#25341=CARTESIAN_POINT('',(1.438300751752,32.3536799039369,214.501561642103));
#25342=CARTESIAN_POINT('Origin',(-69.261699248248,33.853679903937,210.465382311583));
#25343=CARTESIAN_POINT('',(-69.261699248248,33.853679903937,209.965382311583));
#25344=CARTESIAN_POINT('',(-69.261699248248,33.353679903937,210.465382311583));
#25345=CARTESIAN_POINT('Origin',(-69.261699248248,33.853679903937,210.465382311583));
#25346=CARTESIAN_POINT('',(-70.261699248248,33.853679903937,209.965382311583));
#25347=CARTESIAN_POINT('',(-68.061699248248,33.853679903937,209.965382311583));
#25348=CARTESIAN_POINT('',(-70.261699248248,33.353679903937,210.465382311583));
#25349=CARTESIAN_POINT('Origin',(-70.261699248248,33.853679903937,210.465382311583));
#25350=CARTESIAN_POINT('',(-69.261699248248,33.353679903937,210.465382311583));
#25351=CARTESIAN_POINT('Origin',(-68.061699248248,33.853679903937,213.325088768032));
#25352=CARTESIAN_POINT('',(-69.261699248248,33.353679903937,213.325088768032));
#25353=CARTESIAN_POINT('',(-69.261699248248,33.853679903937,213.825088768032));
#25354=CARTESIAN_POINT('Origin',(-69.261699248248,33.853679903937,213.325088768032));
#25355=CARTESIAN_POINT('',(-70.261699248248,33.353679903937,213.325088768032));
#25356=CARTESIAN_POINT('',(-69.261699248248,33.353679903937,213.325088768032));
#25357=CARTESIAN_POINT('',(-70.261699248248,33.853679903937,213.825088768032));
#25358=CARTESIAN_POINT('Origin',(-70.261699248248,33.853679903937,213.325088768032));
#25359=CARTESIAN_POINT('',(-68.061699248248,33.853679903937,213.825088768032));
#25360=CARTESIAN_POINT('Origin',(-68.061699248248,34.553679903937,213.325088768032));
#25361=CARTESIAN_POINT('',(-69.261699248248,34.553679903937,213.825088768032));
#25362=CARTESIAN_POINT('Origin',(-69.261699248248,34.553679903937,213.325088768032));
#25363=CARTESIAN_POINT('',(-70.261699248248,34.553679903937,213.825088768032));
#25364=CARTESIAN_POINT('',(-69.261699248248,34.553679903937,213.825088768032));
#25365=CARTESIAN_POINT('Origin',(-70.261699248248,34.553679903937,213.325088768032));
#25366=CARTESIAN_POINT('',(-70.261699248248,35.053679903937,213.325088768032));
#25367=CARTESIAN_POINT('Origin',(-68.061699248248,34.553679903937,210.465382311583));
#25368=CARTESIAN_POINT('',(-69.261699248248,34.553679903937,209.965382311583));
#25369=CARTESIAN_POINT('Origin',(-69.261699248248,34.553679903937,210.465382311583));
#25370=CARTESIAN_POINT('',(-69.261699248248,35.053679903937,210.465382311583));
#25371=CARTESIAN_POINT('',(-70.261699248248,34.553679903937,209.965382311583));
#25372=CARTESIAN_POINT('Origin',(-70.261699248248,34.553679903937,210.465382311583));
#25373=CARTESIAN_POINT('',(-70.261699248248,34.553679903937,209.965382311583));
#25374=CARTESIAN_POINT('Origin',(-69.261699248248,33.353679903937,215.5));
#25375=CARTESIAN_POINT('',(-70.261699248248,33.353679903937,215.5));
#25376=CARTESIAN_POINT('',(-69.261699248248,32.353679903937,198.5));
#25377=CARTESIAN_POINT('',(-70.261699248248,33.353679903937,215.5));
#25378=CARTESIAN_POINT('',(-70.261699248248,33.353679903937,209.965382311583));
#25379=CARTESIAN_POINT('Origin',(-68.061699248248,35.053679903937,213.825088768032));
#25380=CARTESIAN_POINT('',(-70.261699248248,35.053679903937,213.825088768032));
#25381=CARTESIAN_POINT('',(-69.261699248248,35.553679903937,213.825088768032));
#25382=CARTESIAN_POINT('Origin',(-68.061699248248,35.053679903937,209.965382311583));
#25383=CARTESIAN_POINT('Origin',(-68.061699248248,35.053679903937,209.965382311583));
#25384=CARTESIAN_POINT('',(-69.261699248248,35.553679903937,209.965382311583));
#25385=CARTESIAN_POINT('',(-70.261699248248,35.053679903937,209.965382311583));
#25386=CARTESIAN_POINT('Origin',(-69.261699248248,35.553679903937,209.3));
#25387=CARTESIAN_POINT('',(-69.261699248248,33.353679903937,209.3));
#25388=CARTESIAN_POINT('Origin',(-70.261699248248,33.353679903937,215.5));
#25389=CARTESIAN_POINT('Origin',(-70.261699248248,33.353679903937,214.5));
#25390=CARTESIAN_POINT('',(-69.261699248248,33.353679903937,214.5));
#25391=CARTESIAN_POINT('',(-69.261699248248,33.353679903937,214.5));
#25392=CARTESIAN_POINT('',(-69.261699248248,33.353679903937,214.5));
#25393=CARTESIAN_POINT('Origin',(-70.261699248248,33.353679903937,209.3));
#25394=CARTESIAN_POINT('',(-69.261699248248,33.353679903937,209.3));
#25395=CARTESIAN_POINT('',(-69.261699248248,33.353679903937,209.3));
#25396=CARTESIAN_POINT('',(-69.261699248248,33.353679903937,209.3));
#25397=CARTESIAN_POINT('Origin',(-64.261699248248,32.2748332073223,212.5));
#25398=CARTESIAN_POINT('',(-35.261699248248,32.2748332073222,214.210180047071));
#25399=CARTESIAN_POINT('',(-64.261699248248,32.2748332073223,214.210180047071));
#25400=CARTESIAN_POINT('',(-69.261699248248,32.2748332073223,214.210180047071));
#25401=CARTESIAN_POINT('',(-64.261699248248,32.2748332073223,215.5));
#25402=CARTESIAN_POINT('',(-64.261699248248,32.2748332073223,212.5));
#25403=CARTESIAN_POINT('',(-35.261699248248,32.2748332073222,215.5));
#25404=CARTESIAN_POINT('',(-64.261699248248,32.2748332073223,215.5));
#25405=CARTESIAN_POINT('',(-35.261699248248,32.2748332073222,212.5));
#25406=CARTESIAN_POINT('Origin',(-35.261699248248,33.7748332073222,212.5));
#25407=CARTESIAN_POINT('',(-35.261699248248,33.353679903937,214.5));
#25408=CARTESIAN_POINT('Origin',(-35.261699248248,31.72644166258,213.826414496105));
#25409=CARTESIAN_POINT('',(-35.261699248248,33.353679903937,214.5));
#25410=CARTESIAN_POINT('',(-35.261699248248,32.353679903937,214.095949172));
#25411=CARTESIAN_POINT('',(-35.261699248248,32.353679903937,198.5));
#25412=CARTESIAN_POINT('Origin',(-35.261699248248,30.5438127434663,212.93103382282));
#25413=CARTESIAN_POINT('Origin',(-64.261699248248,33.7748332073223,212.5));
#25414=CARTESIAN_POINT('Origin',(-64.261699248248,30.5438127434664,212.93103382282));
#25415=CARTESIAN_POINT('',(-64.261699248248,32.353679903937,198.5));
#25416=CARTESIAN_POINT('',(-64.261699248248,33.353679903937,214.5));
#25417=CARTESIAN_POINT('',(-64.261699248248,33.353679903937,214.5));
#25418=CARTESIAN_POINT('Origin',(-64.261699248248,31.72644166258,213.826414496105));
#25419=CARTESIAN_POINT('Origin',(-32.261699248248,32.2748332073222,212.5));
#25420=CARTESIAN_POINT('',(-16.261699248248,32.2748332073222,214.210180047071));
#25421=CARTESIAN_POINT('',(-32.261699248248,32.2748332073222,214.210180047071));
#25422=CARTESIAN_POINT('',(-69.261699248248,32.2748332073223,214.210180047071));
#25423=CARTESIAN_POINT('',(-32.261699248248,32.2748332073222,215.5));
#25424=CARTESIAN_POINT('',(-32.261699248248,32.2748332073222,212.5));
#25425=CARTESIAN_POINT('',(-16.261699248248,32.2748332073222,215.5));
#25426=CARTESIAN_POINT('',(-32.261699248248,32.2748332073222,215.5));
#25427=CARTESIAN_POINT('',(-16.261699248248,32.2748332073222,212.5));
#25428=CARTESIAN_POINT('Origin',(-16.261699248248,32.2748332073222,212.5));
#25429=CARTESIAN_POINT('',(-16.261699248248,33.353679903937,214.5));
#25430=CARTESIAN_POINT('Origin',(-16.261699248248,31.72644166258,213.826414496105));
#25431=CARTESIAN_POINT('',(-16.261699248248,33.353679903937,214.5));
#25432=CARTESIAN_POINT('',(-16.261699248248,32.353679903937,214.095949172));
#25433=CARTESIAN_POINT('',(-16.261699248248,32.353679903937,198.5));
#25434=CARTESIAN_POINT('Origin',(-16.261699248248,30.5438127434663,212.93103382282));
#25435=CARTESIAN_POINT('Origin',(-32.261699248248,32.2748332073222,212.5));
#25436=CARTESIAN_POINT('',(-32.261699248248,32.353679903937,214.095949172));
#25437=CARTESIAN_POINT('',(-32.261699248248,32.353679903937,214.471369141518));
#25438=CARTESIAN_POINT('',(-32.261699248248,33.353679903937,214.5));
#25439=CARTESIAN_POINT('',(-32.261699248248,33.353679903937,214.5));
#25440=CARTESIAN_POINT('Origin',(-32.261699248248,31.72644166258,213.826414496105));
#25441=CARTESIAN_POINT('Origin',(-32.261699248248,30.5438127434663,212.93103382282));
#25442=CARTESIAN_POINT('Origin',(-65.261699248248,27.1079166291735,201.645652141467));
#25443=CARTESIAN_POINT('',(-66.861699248248,27.1079166291735,214.5));
#25444=CARTESIAN_POINT('',(-66.861699248248,27.1079166291735,215.5));
#25445=CARTESIAN_POINT('',(-66.861699248248,27.1079166291735,201.645652141467));
#25446=CARTESIAN_POINT('',(-63.661699248248,27.1079166291735,215.5));
#25447=CARTESIAN_POINT('Origin',(-65.261699248248,27.1079166291735,215.5));
#25448=CARTESIAN_POINT('',(-63.661699248248,27.1079166291735,214.5));
#25449=CARTESIAN_POINT('',(-63.661699248248,27.1079166291735,201.645652141467));
#25450=CARTESIAN_POINT('Origin',(-65.261699248248,27.1079166291735,214.5));
#25451=CARTESIAN_POINT('Origin',(-66.861699248248,27.1079166291735,201.645652141467));
#25452=CARTESIAN_POINT('',(-66.861699248248,29.6079166291735,214.5));
#25453=CARTESIAN_POINT('',(-66.861699248248,29.6079166291735,215.5));
#25454=CARTESIAN_POINT('',(-66.861699248248,29.6079166291735,201.645652141467));
#25455=CARTESIAN_POINT('',(-66.861699248248,27.1079166291735,215.5));
#25456=CARTESIAN_POINT('',(-66.861699248248,27.1079166291735,214.5));
#25457=CARTESIAN_POINT('Origin',(-65.261699248248,29.6079166291735,201.645652141467));
#25458=CARTESIAN_POINT('',(-63.661699248248,29.6079166291735,214.5));
#25459=CARTESIAN_POINT('',(-63.661699248248,29.6079166291735,215.5));
#25460=CARTESIAN_POINT('',(-63.661699248248,29.6079166291735,201.645652141467));
#25461=CARTESIAN_POINT('Origin',(-65.261699248248,29.6079166291735,215.5));
#25462=CARTESIAN_POINT('Origin',(-65.261699248248,29.6079166291735,214.5));
#25463=CARTESIAN_POINT('Origin',(-63.661699248248,27.1079166291735,201.645652141467));
#25464=CARTESIAN_POINT('',(-63.661699248248,27.1079166291735,215.5));
#25465=CARTESIAN_POINT('',(-63.661699248248,27.1079166291735,214.5));
#25466=CARTESIAN_POINT('Origin',(-11.261699248248,27.1079166291735,201.645652141467));
#25467=CARTESIAN_POINT('',(-12.861699248248,27.1079166291735,214.5));
#25468=CARTESIAN_POINT('',(-12.861699248248,27.1079166291735,215.5));
#25469=CARTESIAN_POINT('',(-12.861699248248,27.1079166291735,201.645652141467));
#25470=CARTESIAN_POINT('',(-9.66169924824801,27.1079166291735,215.5));
#25471=CARTESIAN_POINT('Origin',(-11.261699248248,27.1079166291735,215.5));
#25472=CARTESIAN_POINT('',(-9.66169924824801,27.1079166291735,214.5));
#25473=CARTESIAN_POINT('',(-9.66169924824804,27.1079166291735,201.645652141467));
#25474=CARTESIAN_POINT('Origin',(-11.261699248248,27.1079166291735,214.5));
#25475=CARTESIAN_POINT('Origin',(-12.861699248248,27.1079166291735,201.645652141467));
#25476=CARTESIAN_POINT('',(-12.861699248248,29.6079166291735,214.5));
#25477=CARTESIAN_POINT('',(-12.861699248248,29.6079166291735,215.5));
#25478=CARTESIAN_POINT('',(-12.861699248248,29.6079166291735,201.645652141467));
#25479=CARTESIAN_POINT('',(-12.861699248248,27.1079166291735,215.5));
#25480=CARTESIAN_POINT('',(-12.861699248248,27.1079166291735,214.5));
#25481=CARTESIAN_POINT('Origin',(-11.261699248248,29.6079166291735,201.645652141467));
#25482=CARTESIAN_POINT('',(-9.66169924824801,29.6079166291735,214.5));
#25483=CARTESIAN_POINT('',(-9.66169924824801,29.6079166291735,215.5));
#25484=CARTESIAN_POINT('',(-9.66169924824804,29.6079166291735,201.645652141467));
#25485=CARTESIAN_POINT('Origin',(-11.261699248248,29.6079166291735,215.5));
#25486=CARTESIAN_POINT('Origin',(-11.261699248248,29.6079166291735,214.5));
#25487=CARTESIAN_POINT('Origin',(-9.66169924824804,27.1079166291735,201.645652141467));
#25488=CARTESIAN_POINT('',(-9.66169924824801,27.1079166291735,215.5));
#25489=CARTESIAN_POINT('',(-9.66169924824801,27.1079166291735,214.5));
#25490=CARTESIAN_POINT('Origin',(-7.26169924824804,24.053679903937,201.645652141467));
#25491=CARTESIAN_POINT('',(-7.261699248248,33.3536799039369,214.5));
#25492=CARTESIAN_POINT('',(-7.261699248248,32.2748332073222,215.5));
#25493=CARTESIAN_POINT('Origin',(-7.26169924824801,31.72644166258,213.826414496105));
#25494=CARTESIAN_POINT('',(-7.26169924824801,24.053679903937,215.5));
#25495=CARTESIAN_POINT('',(-7.26169924824801,24.053679903937,215.5));
#25496=CARTESIAN_POINT('',(-7.26169924824802,24.053679903937,214.5));
#25497=CARTESIAN_POINT('',(-7.26169924824804,24.053679903937,201.645652141467));
#25498=CARTESIAN_POINT('',(-7.261699248248,32.0172414129883,214.5));
#25499=CARTESIAN_POINT('',(-7.26169924824802,24.053679903937,214.5));
#25500=CARTESIAN_POINT('',(-7.26169924824802,24.053679903937,214.5));
#25501=CARTESIAN_POINT('Origin',(-69.261699248248,32.0172414129883,214.5));
#25502=CARTESIAN_POINT('',(-69.261699248248,33.353679903937,214.5));
#25503=CARTESIAN_POINT('',(1.438300751752,32.0172414129883,214.5));
#25504=CARTESIAN_POINT('',(-69.261699248248,32.0172414129883,214.5));
#25505=CARTESIAN_POINT('',(1.43830075175199,31.72644166258,214.5));
#25506=CARTESIAN_POINT('Origin',(1.43830075175199,31.72644166258,213.826414496105));
#25507=CARTESIAN_POINT('',(1.43830075175199,32.3536799039369,214.095949171999));
#25508=CARTESIAN_POINT('',(1.438300751752,32.3536799039369,214.501561642103));
#25509=CARTESIAN_POINT('Origin',(1.43830075175199,30.5438127434663,212.93103382282));
#25510=CARTESIAN_POINT('Origin',(-69.261699248248,32.0172414129883,214.5));
#25511=CARTESIAN_POINT('',(-69.261699248248,24.053679903937,214.5));
#25512=CARTESIAN_POINT('',(-69.261699248248,24.053679903937,214.5));
#25513=CARTESIAN_POINT('',(-69.261699248248,32.0172414129883,214.5));
#25514=CARTESIAN_POINT('',(-69.261699248248,32.0172414129883,214.5));
#25515=CARTESIAN_POINT('',(-69.261699248248,32.0172414129883,214.5));
#25516=CARTESIAN_POINT('Origin',(-69.261699248248,30.5438127434664,212.93103382282));
#25517=CARTESIAN_POINT('',(-69.261699248248,32.353679903937,214.095949172));
#25518=CARTESIAN_POINT('',(-69.261699248248,32.353679903937,214.095949172));
#25519=CARTESIAN_POINT('Origin',(-69.261699248248,30.5438127434664,212.93103382282));
#25520=CARTESIAN_POINT('Origin',(-69.261699248248,32.353679903937,198.5));
#25521=CARTESIAN_POINT('',(-69.261699248248,32.353679903937,198.5));
#25522=CARTESIAN_POINT('',(-69.261699248248,32.353679903937,198.5));
#25523=CARTESIAN_POINT('',(-69.261699248248,32.353679903937,198.5));
#25524=CARTESIAN_POINT('',(1.43830075175196,32.3536799039369,198.5));
#25525=CARTESIAN_POINT('',(-32.261699248248,32.353679903937,198.5));
#25526=CARTESIAN_POINT('Origin',(-69.261699248248,33.353679903937,198.5));
#25527=CARTESIAN_POINT('',(-69.261699248248,33.353679903937,198.5));
#25528=CARTESIAN_POINT('',(-69.261699248248,33.353679903937,198.5));
#25529=CARTESIAN_POINT('',(-69.261699248248,33.353679903937,198.5));
#25530=CARTESIAN_POINT('Origin',(-69.261699248248,33.353679903937,214.5));
#25531=CARTESIAN_POINT('',(-32.261699248248,33.353679903937,214.5));
#25532=CARTESIAN_POINT('',(-69.261699248248,33.353679903937,214.5));
#25533=CARTESIAN_POINT('',(1.438300751752,33.3536799039369,214.5));
#25534=CARTESIAN_POINT('',(-69.261699248248,33.353679903937,214.5));
#25535=CARTESIAN_POINT('',(-69.261699248248,33.353679903937,209.3));
#25536=CARTESIAN_POINT('',(-69.261699248248,33.353679903937,214.5));
#25537=CARTESIAN_POINT('',(-69.261699248248,33.353679903937,214.5));
#25538=CARTESIAN_POINT('Origin',(-69.261699248248,31.72644166258,213.826414496105));
#25539=CARTESIAN_POINT('',(-69.261699248248,32.2748332073223,215.5));
#25540=CARTESIAN_POINT('Origin',(-69.261699248248,24.053679903937,215.5));
#25541=CARTESIAN_POINT('',(-69.261699248248,32.2748332073223,215.5));
#25542=CARTESIAN_POINT('',(-69.261699248248,32.2748332073223,215.5));
#25543=CARTESIAN_POINT('',(-69.261699248248,32.2748332073223,215.5));
#25544=CARTESIAN_POINT('',(-69.261699248248,24.053679903937,215.5));
#25545=CARTESIAN_POINT('',(-69.261699248248,24.053679903937,215.5));
#25546=CARTESIAN_POINT('',(-69.261699248248,24.053679903937,215.5));
#25547=CARTESIAN_POINT('Origin',(-69.261699248248,24.053679903937,214.5));
#25548=CARTESIAN_POINT('',(-69.261699248248,24.053679903937,214.5));
#25549=CARTESIAN_POINT('Origin',(-69.261699248248,31.72644166258,213.826414496105));
#25550=CARTESIAN_POINT('Origin',(-69.261699248248,31.72644166258,213.826414496105));
#25551=CARTESIAN_POINT('Origin',(-69.261699248248,31.72644166258,213.826414496105));
#25552=CARTESIAN_POINT('Origin',(-69.261699248248,31.72644166258,213.826414496105));
#25553=CARTESIAN_POINT('Origin',(-69.261699248248,31.72644166258,213.826414496105));
#25554=CARTESIAN_POINT('Origin',(1.43830075175199,31.72644166258,213.826414496105));
#25555=CARTESIAN_POINT('Origin',(-32.261699248248,32.2748332073222,212.5));
#25556=CARTESIAN_POINT('Origin',(-70.261699248248,33.353679903937,215.5));
#25557=CARTESIAN_POINT('Origin',(-69.261699248248,35.553679903937,209.3));
#36647=UNCERTAINTY_MEASURE_WITH_UNIT(LENGTH_MEASURE(0.01),#36669,
'DISTANCE_ACCURACY_VALUE',
'Maximum model space distance between geometric entities at asserted c
onnectivities');
#36656=UNCERTAINTY_MEASURE_WITH_UNIT(LENGTH_MEASURE(0.01),#36669,
'DISTANCE_ACCURACY_VALUE',
'Maximum model space distance between geometric entities at asserted c
onnectivities');
#36659=(
GEOMETRIC_REPRESENTATION_CONTEXT(3)
GLOBAL_UNCERTAINTY_ASSIGNED_CONTEXT((#36647))
GLOBAL_UNIT_ASSIGNED_CONTEXT((#36669,#36671,#36672))
REPRESENTATION_CONTEXT('','3D')
);
#36668=(
GEOMETRIC_REPRESENTATION_CONTEXT(3)
GLOBAL_UNCERTAINTY_ASSIGNED_CONTEXT((#36656))
GLOBAL_UNIT_ASSIGNED_CONTEXT((#36669,#36671,#36672))
REPRESENTATION_CONTEXT('','3D')
);
#36669=(
LENGTH_UNIT()
NAMED_UNIT(*)
SI_UNIT(.MILLI.,.METRE.)
);
#36671=(
NAMED_UNIT(*)
PLANE_ANGLE_UNIT()
SI_UNIT($,.RADIAN.)
);
#36672=(
NAMED_UNIT(*)
SI_UNIT($,.STERADIAN.)
SOLID_ANGLE_UNIT()
);
#36675=SHAPE_DEFINITION_REPRESENTATION(#36686,#36707);
#36686=PRODUCT_DEFINITION_SHAPE('',$,#36719);
#36707=SHAPE_REPRESENTATION('',(#18105),#36659);
#36716=PRODUCT_DEFINITION_CONTEXT('part definition',#36751,'design');
#36719=PRODUCT_DEFINITION('Component Pick Up Window Plate',
'Component Pick Up Window Plate',#36730,#36716);
#36730=PRODUCT_DEFINITION_FORMATION('',$,#36755);
#36751=APPLICATION_CONTEXT(
'Core Data for Automotive Mechanical Design Process');
#36752=PRODUCT_CONTEXT('part definition',#36751,'mechanical');
#36755=PRODUCT('Component Pick Up Window Plate',
'Component Pick Up Window Plate',$,(#36752));
#36766=PRESENTATION_STYLE_ASSIGNMENT((#36773));
#36773=SURFACE_STYLE_USAGE(.BOTH.,#36780);
#36780=SURFACE_SIDE_STYLE('',(#36787));
#36787=SURFACE_STYLE_FILL_AREA(#36794);
#36794=FILL_AREA_STYLE('Opaque(104,114,127)',(#36801));
#36801=FILL_AREA_STYLE_COLOUR('Opaque(104,114,127)',#36808);
#36808=COLOUR_RGB('Opaque(104,114,127)',0.407843137254902,0.447058823529412,
0.498039215686275);
ENDSEC;
END-ISO-10303-21;
